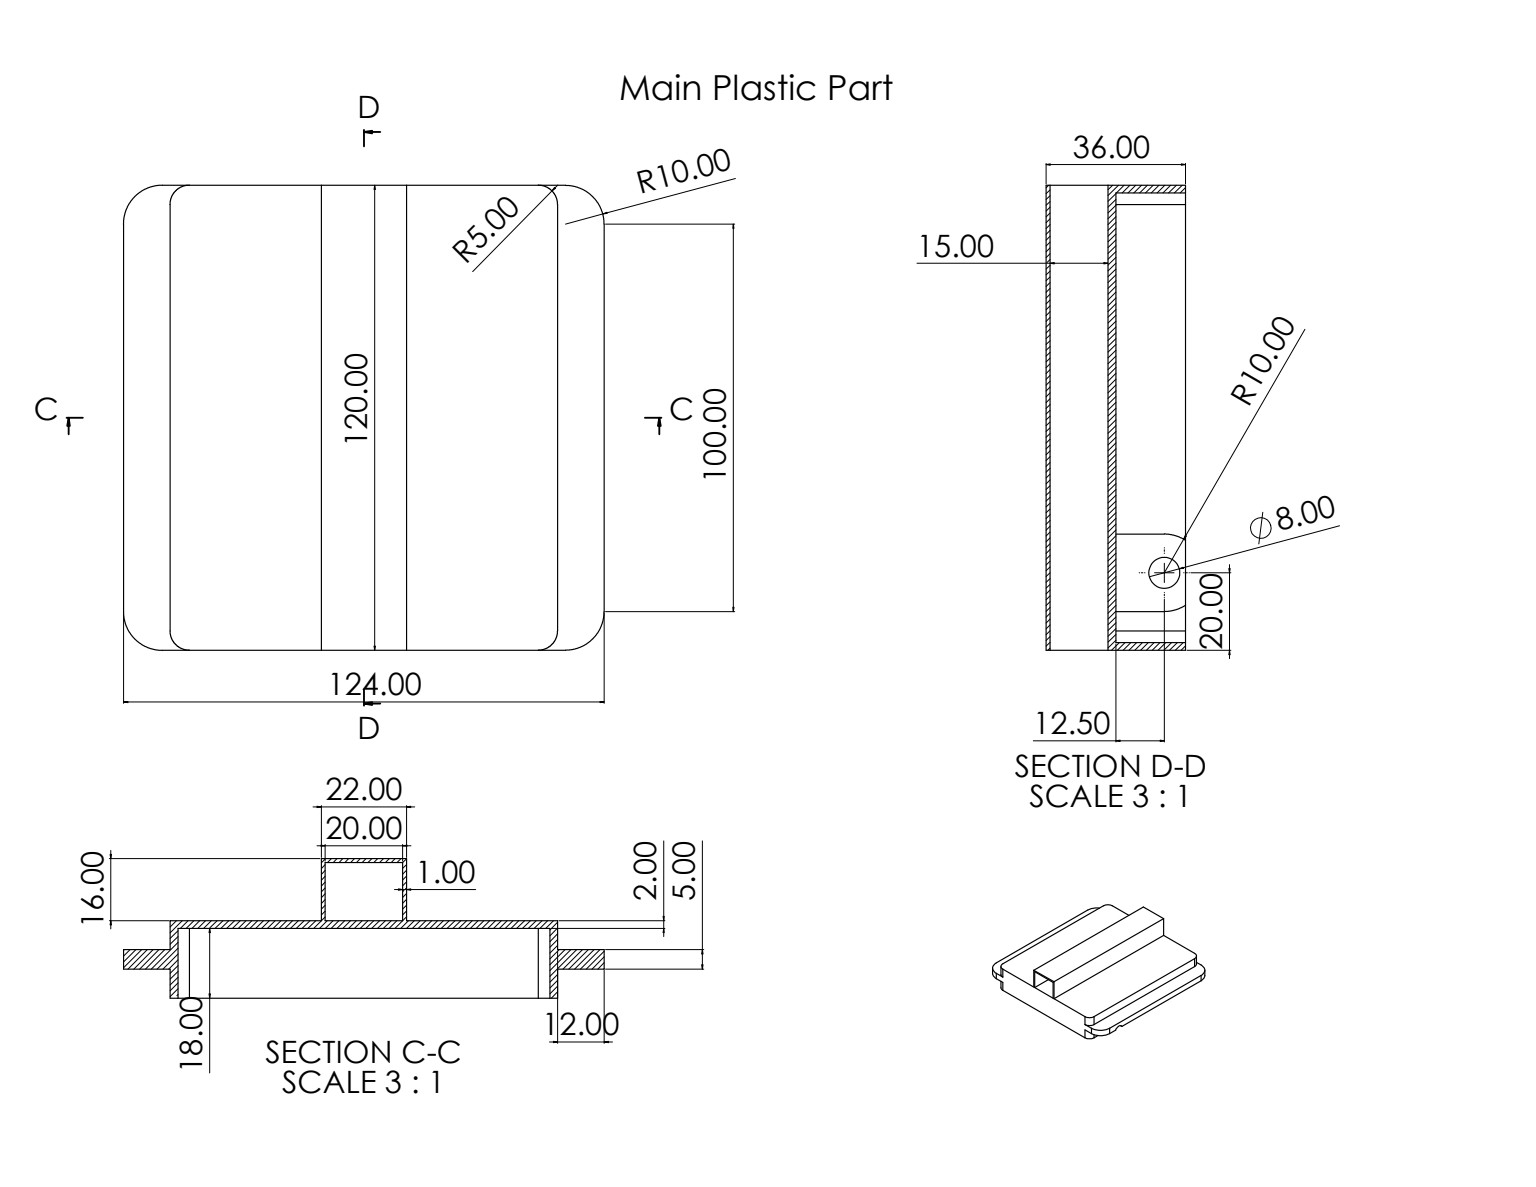
ISO-10303-21;
HEADER;
FILE_DESCRIPTION (('STEP AP214'),
    '1' );
FILE_NAME ('Main Plastic Part.step',
    '2026-10-25T21:42:00',
    ( '' ),
    ( '' ),
    'SwSTEP 2.0',
    'SolidWorks 2025',
    '' );
FILE_SCHEMA (( 'AUTOMOTIVE_DESIGN' ));
ENDSEC;

DATA;
#11=EDGE_CURVE ( 'NONE', #40605, #21661, #7711, .T. ) ;
#16=ORIENTED_EDGE ( 'NONE', *, *, #15282, .F. ) ;
#30=DIRECTION ( 'NONE',  ( 0.000000000000000000, 0.000000000000000000, -1.000000000000000000 ) ) ;
#37=ORIENTED_EDGE ( 'NONE', *, *, #25177, .T. ) ;
#107=ORIENTED_EDGE ( 'NONE', *, *, #6079, .F. ) ;
#112=DIRECTION ( 'NONE',  ( 1.000000000000000000, -0.000000000000000000, -1.067522139062650178E-16 ) ) ;
#115=ORIENTED_EDGE ( 'NONE', *, *, #15723, .T. ) ;
#159=DIRECTION ( 'NONE',  ( 0.000000000000000000, 0.000000000000000000, -1.000000000000000000 ) ) ;
#164=DIRECTION ( 'NONE',  ( -1.000000000000000000, -0.000000000000000000, -0.000000000000000000 ) ) ;
#179=CARTESIAN_POINT ( 'NONE',  ( 10.00000000000000178, 25.00000000000000000, -59.99999999999999289 ) ) ;
#204=ADVANCED_FACE ( 'NONE', ( #16223 ), #3440, .F. ) ;
#231=CARTESIAN_POINT ( 'NONE',  ( 43.18024297220213015, -8.265739277488476588, 38.63781537048668469 ) ) ;
#235=CARTESIAN_POINT ( 'NONE',  ( -50.00000000000001421, -10.00000000000000000, 55.00000000000002132 ) ) ;
#246=DIRECTION ( 'NONE',  ( -0.000000000000000000, -1.000000000000000000, 0.000000000000000000 ) ) ;
#261=ORIENTED_EDGE ( 'NONE', *, *, #37253, .F. ) ;
#327=VECTOR ( 'NONE', #3330, 1000.000000000000000 ) ;
#328=ORIENTED_EDGE ( 'NONE', *, *, #28458, .T. ) ;
#341=PRODUCT_DEFINITION_CONTEXT ( 'detailed design', #12504, 'design' ) ;
#348=CARTESIAN_POINT ( 'NONE',  ( 33.00000000000001421, -10.00000000000000000, 48.35164654424506381 ) ) ;
#443=CARTESIAN_POINT ( 'NONE',  ( 43.17447727835383375, -8.261632567776716840, 41.37333478126254960 ) ) ;
#464=DIRECTION ( 'NONE',  ( 0.000000000000000000, 0.000000000000000000, -1.000000000000000000 ) ) ;
#496=CYLINDRICAL_SURFACE ( 'NONE', #39467, 4.000000000000003553 ) ;
#556=LINE ( 'NONE', #37343, #4887 ) ;
#564=CARTESIAN_POINT ( 'NONE',  ( -62.00000000000002842, -2.499999999999999556, 43.46410161513779258 ) ) ;
#592=ORIENTED_EDGE ( 'NONE', *, *, #4818, .T. ) ;
#604=CARTESIAN_POINT ( 'NONE',  ( 0.000000000000000000, 8.000000000000000000, 0.000000000000000000 ) ) ;
#625=CARTESIAN_POINT ( 'NONE',  ( -62.00000000000002842, -4.500000000000000000, 40.00000000000002842 ) ) ;
#626=VERTEX_POINT ( 'NONE', #3867 ) ;
#638=VECTOR ( 'NONE', #26031, 1000.000000000000000 ) ;
#646=EDGE_CURVE ( 'NONE', #32443, #25917, #5124, .T. ) ;
#653=CARTESIAN_POINT ( 'NONE',  ( 40.70800149128672274, -7.145751311064596933, 37.00000000000002132 ) ) ;
#657=AXIS2_PLACEMENT_3D ( 'NONE', #29066, #36076, #42060 ) ;
#680=LINE ( 'NONE', #26634, #18481 ) ;
#687=DIRECTION ( 'NONE',  ( 1.000000000000000000, 0.000000000000000000, -0.000000000000000000 ) ) ;
#693=ORIENTED_EDGE ( 'NONE', *, *, #31287, .T. ) ;
#729=CARTESIAN_POINT ( 'NONE',  ( 39.50407584885977741, -7.322325674842114829, 42.83643345649426948 ) ) ;
#740=ORIENTED_EDGE ( 'NONE', *, *, #15093, .T. ) ;
#746=VERTEX_POINT ( 'NONE', #11497 ) ;
#774=DIRECTION ( 'NONE',  ( -0.000000000000000000, -0.000000000000000000, 1.000000000000000000 ) ) ;
#779=DIRECTION ( 'NONE',  ( 0.000000000000000000, -1.000000000000000000, 0.000000000000000000 ) ) ;
#795=EDGE_CURVE ( 'NONE', #21937, #903, #18515, .T. ) ;
#798=DIRECTION ( 'NONE',  ( 0.000000000000000000, 0.000000000000000000, -1.000000000000000000 ) ) ;
#806=DIRECTION ( 'NONE',  ( 0.000000000000000000, 1.000000000000000000, 0.000000000000000000 ) ) ;
#808=ORIENTED_EDGE ( 'NONE', *, *, #26182, .F. ) ;
#831=FACE_OUTER_BOUND ( 'NONE', #36369, .T. ) ;
#836=EDGE_LOOP ( 'NONE', ( #19778, #12521, #31733, #1428 ) ) ;
#864=ORIENTED_EDGE ( 'NONE', *, *, #5050, .T. ) ;
#875=AXIS2_PLACEMENT_3D ( 'NONE', #35943, #32748, #35537 ) ;
#895=VERTEX_POINT ( 'NONE', #14657 ) ;
#903=VERTEX_POINT ( 'NONE', #30600 ) ;
#910=VECTOR ( 'NONE', #30254, 1000.000000000000000 ) ;
#912=CARTESIAN_POINT ( 'NONE',  ( -50.00000000000001421, -4.500000000000000000, 40.00000000000002842 ) ) ;
#932=ADVANCED_FACE ( 'NONE', ( #5066, #11042 ), #8259, .F. ) ;
#949=CARTESIAN_POINT ( 'NONE',  ( 38.25871219653468813, -7.965888518254534034, 37.99698286429647709 ) ) ;
#957=ORIENTED_EDGE ( 'NONE', *, *, #37845, .T. ) ;
#962=ORIENTED_EDGE ( 'NONE', *, *, #32421, .T. ) ;
#1024=ORIENTED_EDGE ( 'NONE', *, *, #38610, .T. ) ;
#1025=VERTEX_POINT ( 'NONE', #18250 ) ;
#1029=DIRECTION ( 'NONE',  ( -1.000000000000000000, 0.000000000000000000, 1.067522139062650178E-16 ) ) ;
#1030=EDGE_CURVE ( 'NONE', #9283, #5870, #25406, .T. ) ;
#1040=AXIS2_PLACEMENT_3D ( 'NONE', #31418, #28431, #21630 ) ;
#1104=FACE_OUTER_BOUND ( 'NONE', #28266, .T. ) ;
#1165=FACE_OUTER_BOUND ( 'NONE', #24935, .T. ) ;
#1172=ORIENTED_EDGE ( 'NONE', *, *, #25644, .F. ) ;
#1179=VERTEX_POINT ( 'NONE', #29916 ) ;
#1210=DIRECTION ( 'NONE',  ( 0.000000000000000000, -1.000000000000000000, 0.000000000000000000 ) ) ;
#1211=VERTEX_POINT ( 'NONE', #23115 ) ;
#1217=CARTESIAN_POINT ( 'NONE',  ( -73.31370849898480913, -2.499999999999999556, 36.53589838486226427 ) ) ;
#1223=ORIENTED_EDGE ( 'NONE', *, *, #11786, .T. ) ;
#1232=DIRECTION ( 'NONE',  ( 1.000000000000000000, -0.000000000000000000, 1.156482317317871232E-16 ) ) ;
#1234=ADVANCED_FACE ( 'NONE', ( #19714 ), #38865, .T. ) ;
#1240=AXIS2_PLACEMENT_3D ( 'NONE', #3587, #9987, #2755 ) ;
#1262=EDGE_CURVE ( 'NONE', #27592, #25543, #32683, .T. ) ;
#1265=LINE ( 'NONE', #17638, #24662 ) ;
#1273=DIRECTION ( 'NONE',  ( -1.000000000000000000, 0.000000000000000000, 0.000000000000000000 ) ) ;
#1285=AXIS2_PLACEMENT_3D ( 'NONE', #6696, #16904, #26478 ) ;
#1318=ORIENTED_EDGE ( 'NONE', *, *, #17030, .F. ) ;
#1333=ORIENTED_EDGE ( 'NONE', *, *, #37843, .T. ) ;
#1355=FACE_OUTER_BOUND ( 'NONE', #24355, .T. ) ;
#1363=ORIENTED_EDGE ( 'NONE', *, *, #20185, .T. ) ;
#1366=DIRECTION ( 'NONE',  ( 0.000000000000000000, -1.000000000000000000, 0.000000000000000000 ) ) ;
#1367=CARTESIAN_POINT ( 'NONE',  ( 38.25522726963416176, -7.968137130668702994, 41.99918083815303760 ) ) ;
#1378=ORIENTED_EDGE ( 'NONE', *, *, #10228, .F. ) ;
#1380=VECTOR ( 'NONE', #12567, 1000.000000000000000 ) ;
#1404=CARTESIAN_POINT ( 'NONE',  ( -50.00000000000001421, -10.00000000000000000, -59.99999999999999289 ) ) ;
#1428=ORIENTED_EDGE ( 'NONE', *, *, #13150, .T. ) ;
#1429=VERTEX_POINT ( 'NONE', #23010 ) ;
#1442=CARTESIAN_POINT ( 'NONE',  ( -11.00000000000000355, 26.00000000000000355, -87.20294101747086302 ) ) ;
#1449=VECTOR ( 'NONE', #35176, 1000.000000000000000 ) ;
#1458=CARTESIAN_POINT ( 'NONE',  ( 10.00000000000000178, 10.00000000000000000, -87.20294101747086302 ) ) ;
#1462=CARTESIAN_POINT ( 'NONE',  ( -50.00000000000001421, -10.00000000000000000, 60.00000000000002132 ) ) ;
#1487=CARTESIAN_POINT ( 'NONE',  ( 11.00000000000000355, 26.00000000000000355, 60.00000000000002132 ) ) ;
#1489=EDGE_CURVE ( 'NONE', #27620, #7819, #28127, .T. ) ;
#1495=VECTOR ( 'NONE', #26536, 1000.000000000000000 ) ;
#1517=VECTOR ( 'NONE', #35936, 1000.000000000000000 ) ;
#1578=CARTESIAN_POINT ( 'NONE',  ( -45.00000000000002132, -10.00000000000000000, 55.00000000000002132 ) ) ;
#1612=AXIS2_PLACEMENT_3D ( 'NONE', #37044, #41057, #34256 ) ;
#1632=VECTOR ( 'NONE', #15338, 1000.000000000000000 ) ;
#1645=VECTOR ( 'NONE', #12236, 1000.000000000000000 ) ;
#1727=DIRECTION ( 'NONE',  ( -0.000000000000000000, 1.000000000000000000, 0.000000000000000000 ) ) ;
#1804=CARTESIAN_POINT ( 'NONE',  ( -73.31370849898480913, -2.499999999999999556, 43.46410161513779258 ) ) ;
#1841=VERTEX_POINT ( 'NONE', #34471 ) ;
#1862=CARTESIAN_POINT ( 'NONE',  ( 0.000000000000000000, -10.00000000000000000, 0.000000000000000000 ) ) ;
#1895=ORIENTED_EDGE ( 'NONE', *, *, #12828, .F. ) ;
#1906=DIRECTION ( 'NONE',  ( 1.000000000000000000, 0.000000000000000000, -1.067522139062650302E-16 ) ) ;
#1945=EDGE_CURVE ( 'NONE', #33276, #24557, #9582, .T. ) ;
#1986=CARTESIAN_POINT ( 'NONE',  ( 10.00000000000000178, 25.00000000000000000, 60.00000000000002132 ) ) ;
#2006=LINE ( 'NONE', #22407, #638 ) ;
#2034=EDGE_CURVE ( 'NONE', #21661, #9431, #36574, .T. ) ;
#2045=EDGE_LOOP ( 'NONE', ( #33378, #14401, #40294, #13987, #23060, #23283, #39786, #27182 ) ) ;
#2069=CARTESIAN_POINT ( 'NONE',  ( 44.99999999999999289, -10.00000000000000000, 55.00000000000002132 ) ) ;
#2087=CARTESIAN_POINT ( 'NONE',  ( 47.99999999999998579, 10.00000000000000000, 55.00000000000002132 ) ) ;
#2100=AXIS2_PLACEMENT_3D ( 'NONE', #11181, #7782, #14788 ) ;
#2110=ORIENTED_EDGE ( 'NONE', *, *, #28530, .T. ) ;
#2134=CARTESIAN_POINT ( 'NONE',  ( 52.00000000000002842, 2.499999999999999556, 50.00000000000001421 ) ) ;
#2137=DIRECTION ( 'NONE',  ( -1.000000000000000000, 0.000000000000000000, 0.000000000000000000 ) ) ;
#2148=CARTESIAN_POINT ( 'NONE',  ( -48.00000000000001421, 8.000000000000000000, 55.00000000000002132 ) ) ;
#2161=ORIENTED_EDGE ( 'NONE', *, *, #14749, .T. ) ;
#2180=DIRECTION ( 'NONE',  ( 0.000000000000000000, 0.000000000000000000, -1.000000000000000000 ) ) ;
#2206=AXIS2_PLACEMENT_3D ( 'NONE', #34511, #5369, #18348 ) ;
#2215=CARTESIAN_POINT ( 'NONE',  ( 40.50000000000000711, -15.00000000000000000, 37.00000000000001421 ) ) ;
#2246=ORIENTED_EDGE ( 'NONE', *, *, #5463, .T. ) ;
#2251=DIRECTION ( 'NONE',  ( 1.000000000000000000, -0.000000000000000000, -0.000000000000000000 ) ) ;
#2306=LINE ( 'NONE', #8897, #20278 ) ;
#2317=DIRECTION ( 'NONE',  ( 0.000000000000000000, -0.000000000000000000, 1.000000000000000000 ) ) ;
#2367=FACE_OUTER_BOUND ( 'NONE', #20004, .T. ) ;
#2378=CARTESIAN_POINT ( 'NONE',  ( -45.00000000000002132, 10.00000000000000000, -59.99999999999999289 ) ) ;
#2410=CYLINDRICAL_SURFACE ( 'NONE', #20954, 10.00000000000000178 ) ;
#2431=CARTESIAN_POINT ( 'NONE',  ( 44.99999999999998579, -2.499999999999999556, -60.00000000000000000 ) ) ;
#2449=CARTESIAN_POINT ( 'NONE',  ( -52.00000000000002842, 10.00000000000000000, 50.00000000000001421 ) ) ;
#2466=ADVANCED_FACE ( 'NONE', ( #16576 ), #26563, .T. ) ;
#2475=PLANE ( 'NONE',  #25989 ) ;
#2479=ORIENTED_EDGE ( 'NONE', *, *, #10263, .F. ) ;
#2484=ADVANCED_FACE ( 'NONE', ( #3797 ), #10612, .T. ) ;
#2587=EDGE_CURVE ( 'NONE', #21661, #40605, #5052, .T. ) ;
#2637=AXIS2_PLACEMENT_3D ( 'NONE', #3251, #24973, #19416 ) ;
#2655=DIRECTION ( 'NONE',  ( -0.000000000000000000, -1.000000000000000000, -0.000000000000000000 ) ) ;
#2662=ORIENTED_EDGE ( 'NONE', *, *, #4575, .F. ) ;
#2673=VECTOR ( 'NONE', #26163, 1000.000000000000000 ) ;
#2681=EDGE_LOOP ( 'NONE', ( #33551, #6500, #40081, #37 ) ) ;
#2683=DIRECTION ( 'NONE',  ( -1.000000000000000000, 0.000000000000000000, 0.000000000000000000 ) ) ;
#2688=ORIENTED_EDGE ( 'NONE', *, *, #23153, .T. ) ;
#2700=PLANE ( 'NONE',  #28201 ) ;
#2715=EDGE_LOOP ( 'NONE', ( #328, #26233, #27210, #38333, #36525 ) ) ;
#2716=VECTOR ( 'NONE', #28782, 1000.000000000000000 ) ;
#2725=EDGE_CURVE ( 'NONE', #27773, #37476, #17421, .T. ) ;
#2755=DIRECTION ( 'NONE',  ( 0.000000000000000000, -0.000000000000000000, -1.000000000000000000 ) ) ;
#2769=VERTEX_POINT ( 'NONE', #21018 ) ;
#2789=AXIS2_PLACEMENT_3D ( 'NONE', #41130, #18160, #37931 ) ;
#2794=ORIENTED_EDGE ( 'NONE', *, *, #12455, .T. ) ;
#2825=ORIENTED_EDGE ( 'NONE', *, *, #37937, .F. ) ;
#2828=DIRECTION ( 'NONE',  ( 0.000000000000000000, 0.000000000000000000, -1.000000000000000000 ) ) ;
#2836=ORIENTED_EDGE ( 'NONE', *, *, #40187, .T. ) ;
#2839=ORIENTED_EDGE ( 'NONE', *, *, #2725, .F. ) ;
#2857=DIRECTION ( 'NONE',  ( 1.000000000000000000, -0.000000000000000000, -1.067522139062650178E-16 ) ) ;
#2878=PLANE ( 'NONE',  #12962 ) ;
#2894=FACE_OUTER_BOUND ( 'NONE', #8992, .T. ) ;
#2895=LINE ( 'NONE', #38623, #28106 ) ;
#2907=AXIS2_PLACEMENT_3D ( 'NONE', #17046, #10238, #16835 ) ;
#2971=VECTOR ( 'NONE', #4498, 1000.000000000000000 ) ;
#2990=CARTESIAN_POINT ( 'NONE',  ( -33.00000000000001421, 8.000000000000000000, 50.00000000000002842 ) ) ;
#3019=CARTESIAN_POINT ( 'NONE',  ( 40.50000000000000711, -15.00000000000000000, 40.00000000000002842 ) ) ;
#3101=ORIENTED_EDGE ( 'NONE', *, *, #4888, .T. ) ;
#3104=VERTEX_POINT ( 'NONE', #39473 ) ;
#3107=ORIENTED_EDGE ( 'NONE', *, *, #19744, .T. ) ;
#3118=EDGE_CURVE ( 'NONE', #1025, #28880, #3333, .T. ) ;
#3124=ADVANCED_BREP_SHAPE_REPRESENTATION ( '', ( #10332, #40442 ), #28197 ) ;
#3135=CYLINDRICAL_SURFACE ( 'NONE', #26509, 4.999999999999997335 ) ;
#3142=DIRECTION ( 'NONE',  ( 1.000000000000000000, 0.000000000000000000, -0.000000000000000000 ) ) ;
#3239=DIRECTION ( 'NONE',  ( 0.000000000000000000, -0.000000000000000000, -1.000000000000000000 ) ) ;
#3251=CARTESIAN_POINT ( 'NONE',  ( -50.00000000000001421, 10.00000000000000000, -57.99999999999998579 ) ) ;
#3291=VERTEX_POINT ( 'NONE', #20968 ) ;
#3308=ORIENTED_EDGE ( 'NONE', *, *, #21156, .T. ) ;
#3330=DIRECTION ( 'NONE',  ( -1.156482317317871232E-16, -0.000000000000000000, -1.000000000000000000 ) ) ;
#3333=LINE ( 'NONE', #348, #26173 ) ;
#3357=DIRECTION ( 'NONE',  ( -0.000000000000000000, 1.000000000000000000, -0.000000000000000000 ) ) ;
#3363=FACE_OUTER_BOUND ( 'NONE', #31140, .T. ) ;
#3365=ORIENTED_EDGE ( 'NONE', *, *, #27211, .F. ) ;
#3393=LINE ( 'NONE', #13177, #2673 ) ;
#3402=ORIENTED_EDGE ( 'NONE', *, *, #25736, .T. ) ;
#3423=CARTESIAN_POINT ( 'NONE',  ( 43.47980401598100286, -8.484779524062236788, 39.59649023839028814 ) ) ;
#3440=PLANE ( 'NONE',  #15889 ) ;
#3444=CARTESIAN_POINT ( 'NONE',  ( 44.99999999999999289, 8.000000000000000000, 55.00000000000002132 ) ) ;
#3451=ORIENTED_EDGE ( 'NONE', *, *, #9825, .F. ) ;
#3453=AXIS2_PLACEMENT_3D ( 'NONE', #11912, #21494, #28289 ) ;
#3481=CARTESIAN_POINT ( 'NONE',  ( 62.00000000000002842, -2.499999999999999556, 43.46410161513777837 ) ) ;
#3488=CARTESIAN_POINT ( 'NONE',  ( -45.00000000000002132, 2.499999999999999556, -55.00000000000000000 ) ) ;
#3502=ORIENTED_EDGE ( 'NONE', *, *, #30309, .T. ) ;
#3519=VECTOR ( 'NONE', #774, 1000.000000000000000 ) ;
#3537=FACE_OUTER_BOUND ( 'NONE', #7186, .T. ) ;
#3541=DIRECTION ( 'NONE',  ( 0.000000000000000000, 0.000000000000000000, -1.000000000000000000 ) ) ;
#3572=CARTESIAN_POINT ( 'NONE',  ( -9.999999999999998224, 25.00000000000000000, -59.99999999999999289 ) ) ;
#3587=CARTESIAN_POINT ( 'NONE',  ( 40.50000000000000711, -15.00000000000000000, 40.00000000000002842 ) ) ;
#3630=EDGE_CURVE ( 'NONE', #16152, #5136, #7024, .T. ) ;
#3636=CARTESIAN_POINT ( 'NONE',  ( 49.99999999999998579, 10.00000000000000000, 60.00000000000002132 ) ) ;
#3669=CARTESIAN_POINT ( 'NONE',  ( -52.00000000000002842, -2.500000000000000444, 50.00000000000001421 ) ) ;
#3698=FACE_OUTER_BOUND ( 'NONE', #32650, .T. ) ;
#3718=DIRECTION ( 'NONE',  ( 0.000000000000000000, 0.000000000000000000, 1.000000000000000000 ) ) ;
#3741=DIRECTION ( 'NONE',  ( -0.000000000000000000, -1.000000000000000000, -0.000000000000000000 ) ) ;
#3797=FACE_OUTER_BOUND ( 'NONE', #34218, .T. ) ;
#3799=EDGE_CURVE ( 'NONE', #36692, #33611, #25470, .T. ) ;
#3807=EDGE_CURVE ( 'NONE', #2769, #16441, #13220, .T. ) ;
#3813=DIRECTION ( 'NONE',  ( -1.000000000000000000, 0.000000000000000000, 0.000000000000000000 ) ) ;
#3820=ORIENTED_EDGE ( 'NONE', *, *, #28458, .F. ) ;
#3821=DIRECTION ( 'NONE',  ( -0.000000000000000000, 1.000000000000000000, -0.000000000000000000 ) ) ;
#3829=VERTEX_POINT ( 'NONE', #17468 ) ;
#3847=CARTESIAN_POINT ( 'NONE',  ( 40.50000000000000711, -7.145751311064572064, 43.00000000000004263 ) ) ;
#3867=CARTESIAN_POINT ( 'NONE',  ( -49.99999999999998579, -2.499999999999999556, 43.46410161513779258 ) ) ;
#3884=CARTESIAN_POINT ( 'NONE',  ( -33.00000000000001421, -4.499999999999999112, 44.00000000000003553 ) ) ;
#3926=VERTEX_POINT ( 'NONE', #16167 ) ;
#3936=ORIENTED_EDGE ( 'NONE', *, *, #37619, .F. ) ;
#3956=LINE ( 'NONE', #36284, #3519 ) ;
#3973=CARTESIAN_POINT ( 'NONE',  ( 44.99999999999998579, 2.499999999999999556, 60.00000000000002132 ) ) ;
#3988=ORIENTED_EDGE ( 'NONE', *, *, #15039, .F. ) ;
#4007=CARTESIAN_POINT ( 'NONE',  ( -50.00000000000001421, 10.00000000000000000, 60.00000000000002132 ) ) ;
#4030=VERTEX_POINT ( 'NONE', #5737 ) ;
#4057=CIRCLE ( 'NONE', #16977, 4.000000000000003553 ) ;
#4075=CIRCLE ( 'NONE', #38684, 4.000000000000003553 ) ;
#4121=AXIS2_PLACEMENT_3D ( 'NONE', #36302, #39490, #10579 ) ;
#4126=ADVANCED_FACE ( 'NONE', ( #19969 ), #6577, .F. ) ;
#4135=VERTEX_POINT ( 'NONE', #32936 ) ;
#4205=CARTESIAN_POINT ( 'NONE',  ( -62.00000000000001421, 2.499999999999999556, -60.00000000000000000 ) ) ;
#4209=CARTESIAN_POINT ( 'NONE',  ( -73.31370849898480913, -2.499999999999999556, 43.46410161513779258 ) ) ;
#4217=CIRCLE ( 'NONE', #27986, 10.00000000000000178 ) ;
#4222=DIRECTION ( 'NONE',  ( 0.000000000000000000, -1.000000000000000000, 0.000000000000000000 ) ) ;
#4284=CARTESIAN_POINT ( 'NONE',  ( -33.00000000000001421, -4.500000000000000000, 30.00000000000002842 ) ) ;
#4329=VECTOR ( 'NONE', #2137, 1000.000000000000000 ) ;
#4337=EDGE_CURVE ( 'NONE', #26542, #37769, #27538, .T. ) ;
#4345=CARTESIAN_POINT ( 'NONE',  ( 37.60297877579395021, -8.423259317252886902, 40.80592701207748974 ) ) ;
#4359=ORIENTED_EDGE ( 'NONE', *, *, #40890, .F. ) ;
#4383=CARTESIAN_POINT ( 'NONE',  ( 33.00000000000001421, -4.500000000000000888, 50.00000000000002842 ) ) ;
#4450=CARTESIAN_POINT ( 'NONE',  ( 49.99999999999998579, -2.499999999999999556, -54.99999999999997158 ) ) ;
#4463=ORIENTED_EDGE ( 'NONE', *, *, #1945, .T. ) ;
#4465=CARTESIAN_POINT ( 'NONE',  ( 44.99999999999998579, 2.499999999999999556, -60.00000000000000000 ) ) ;
#4498=DIRECTION ( 'NONE',  ( -0.000000000000000000, -1.000000000000000000, 0.000000000000000000 ) ) ;
#4537=CARTESIAN_POINT ( 'NONE',  ( 47.99999999999998579, 8.000000000000000000, -54.99999999999997158 ) ) ;
#4548=CARTESIAN_POINT ( 'NONE',  ( 49.99999999999998579, 10.00000000000000000, 55.00000000000002132 ) ) ;
#4575=EDGE_CURVE ( 'NONE', #41347, #30811, #12582, .T. ) ;
#4591=CARTESIAN_POINT ( 'NONE',  ( 11.00000000000000355, 26.00000000000000355, -87.20294101747086302 ) ) ;
#4617=ORIENTED_EDGE ( 'NONE', *, *, #36365, .F. ) ;
#4626=CARTESIAN_POINT ( 'NONE',  ( -45.00000000000002132, -2.499999999999999556, 55.00000000000002132 ) ) ;
#4634=EDGE_CURVE ( 'NONE', #26169, #21937, #40928, .T. ) ;
#4651=DIRECTION ( 'NONE',  ( 0.000000000000000000, 0.000000000000000000, -1.000000000000000000 ) ) ;
#4725=EDGE_CURVE ( 'NONE', #2769, #15408, #8600, .T. ) ;
#4775=VECTOR ( 'NONE', #18902, 1000.000000000000000 ) ;
#4782=DIRECTION ( 'NONE',  ( -1.000000000000000000, 0.000000000000000000, 0.000000000000000000 ) ) ;
#4814=ADVANCED_FACE ( 'NONE', ( #15416 ), #28368, .T. ) ;
#4818=EDGE_CURVE ( 'NONE', #21965, #16039, #7982, .T. ) ;
#4822=VERTEX_POINT ( 'NONE', #27553 ) ;
#4854=CARTESIAN_POINT ( 'NONE',  ( -45.00000000000002132, 10.00000000000000000, 60.00000000000002132 ) ) ;
#4869=DIRECTION ( 'NONE',  ( 0.000000000000000000, 0.000000000000000000, -1.000000000000000000 ) ) ;
#4870=VECTOR ( 'NONE', #4222, 1000.000000000000000 ) ;
#4876=ORIENTED_EDGE ( 'NONE', *, *, #41025, .F. ) ;
#4887=VECTOR ( 'NONE', #31159, 1000.000000000000000 ) ;
#4888=EDGE_CURVE ( 'NONE', #13780, #1025, #19868, .T. ) ;
#4895=DIRECTION ( 'NONE',  ( 0.000000000000000000, -1.000000000000000000, 0.000000000000000000 ) ) ;
#4933=CIRCLE ( 'NONE', #29356, 3.000000000000016431 ) ;
#4936=( GEOMETRIC_REPRESENTATION_CONTEXT ( 3 ) GLOBAL_UNCERTAINTY_ASSIGNED_CONTEXT ( ( #22893 ) ) GLOBAL_UNIT_ASSIGNED_CONTEXT ( ( #10878, #34252, #34457 ) ) REPRESENTATION_CONTEXT ( 'NONE', 'WORKASPACE' ) );
#5006=FACE_OUTER_BOUND ( 'NONE', #29572, .T. ) ;
#5009=CARTESIAN_POINT ( 'NONE',  ( -45.00000000000002132, 8.000000000000000000, 55.00000000000002132 ) ) ;
#5028=ORIENTED_EDGE ( 'NONE', *, *, #16775, .T. ) ;
#5050=EDGE_CURVE ( 'NONE', #21937, #9969, #31032, .T. ) ;
#5052=CIRCLE ( 'NONE', #21363, 4.000000000000010658 ) ;
#5060=DIRECTION ( 'NONE',  ( -0.000000000000000000, -0.000000000000000000, 1.000000000000000000 ) ) ;
#5066=FACE_BOUND ( 'NONE', #5614, .T. ) ;
#5069=DIRECTION ( 'NONE',  ( -1.000000000000000000, 0.000000000000000000, 0.000000000000000000 ) ) ;
#5072=DIRECTION ( 'NONE',  ( -0.000000000000000000, 1.000000000000000000, -0.000000000000000000 ) ) ;
#5084=ORIENTED_EDGE ( 'NONE', *, *, #17030, .T. ) ;
#5104=DIRECTION ( 'NONE',  ( 0.000000000000000000, -1.000000000000000000, 0.000000000000000000 ) ) ;
#5124=LINE ( 'NONE', #30657, #4329 ) ;
#5136=VERTEX_POINT ( 'NONE', #12729 ) ;
#5151=CARTESIAN_POINT ( 'NONE',  ( 49.99999999999998579, -10.00000000000000000, 55.00000000000002132 ) ) ;
#5173=APPLICATION_CONTEXT ( 'automotive_design' ) ;
#5201=CARTESIAN_POINT ( 'NONE',  ( 52.00000000000002132, 2.499999999999999556, -60.00000000000000000 ) ) ;
#5222=DIRECTION ( 'NONE',  ( 0.000000000000000000, 0.000000000000000000, -1.000000000000000000 ) ) ;
#5227=ORIENTED_EDGE ( 'NONE', *, *, #5949, .T. ) ;
#5259=ORIENTED_EDGE ( 'NONE', *, *, #38952, .F. ) ;
#5277=ORIENTED_EDGE ( 'NONE', *, *, #8224, .T. ) ;
#5281=CARTESIAN_POINT ( 'NONE',  ( 52.00000000000002132, 10.00000000000000000, 60.00000000000002132 ) ) ;
#5294=VERTEX_POINT ( 'NONE', #26545 ) ;
#5295=CARTESIAN_POINT ( 'NONE',  ( 62.00000000000002842, -2.499999999999999556, 36.53589838486225005 ) ) ;
#5369=DIRECTION ( 'NONE',  ( 0.000000000000000000, -1.000000000000000000, 0.000000000000000000 ) ) ;
#5399=CIRCLE ( 'NONE', #31206, 4.999999999999984013 ) ;
#5421=DIRECTION ( 'NONE',  ( 0.000000000000000000, 0.000000000000000000, 1.000000000000000000 ) ) ;
#5463=EDGE_CURVE ( 'NONE', #36810, #626, #12646, .T. ) ;
#5472=FACE_BOUND ( 'NONE', #38192, .T. ) ;
#5480=CYLINDRICAL_SURFACE ( 'NONE', #657, 10.00000000000000178 ) ;
#5490=LINE ( 'NONE', #21649, #16316 ) ;
#5495=PLANE ( 'NONE',  #29429 ) ;
#5504=VERTEX_POINT ( 'NONE', #27512 ) ;
#5505=AXIS2_PLACEMENT_3D ( 'NONE', #41572, #15628, #31987 ) ;
#5510=EDGE_LOOP ( 'NONE', ( #34428, #8429, #12576, #23384, #26391, #957 ) ) ;
#5514=ORIENTED_EDGE ( 'NONE', *, *, #23156, .F. ) ;
#5523=DIRECTION ( 'NONE',  ( 0.000000000000000000, 0.000000000000000000, -1.000000000000000000 ) ) ;
#5531=CARTESIAN_POINT ( 'NONE',  ( -48.00000000000001421, -10.00000000000000000, 0.000000000000000000 ) ) ;
#5541=CARTESIAN_POINT ( 'NONE',  ( 33.00000000000001421, 7.999999999999996447, 50.00000000000002842 ) ) ;
#5554=ORIENTED_EDGE ( 'NONE', *, *, #4818, .F. ) ;
#5569=VERTEX_POINT ( 'NONE', #4537 ) ;
#5577=AXIS2_PLACEMENT_3D ( 'NONE', #41442, #8680, #40805 ) ;
#5614=EDGE_LOOP ( 'NONE', ( #35753, #962, #592, #7959 ) ) ;
#5622=CARTESIAN_POINT ( 'NONE',  ( 33.00000000000001421, 8.000000000000000000, 30.00000000000002132 ) ) ;
#5635=DIRECTION ( 'NONE',  ( 0.000000000000000000, 0.000000000000000000, -1.000000000000000000 ) ) ;
#5675=DIRECTION ( 'NONE',  ( -1.000000000000000000, -0.000000000000000000, -0.000000000000000000 ) ) ;
#5722=DIRECTION ( 'NONE',  ( 1.000000000000000000, 0.000000000000000000, 0.000000000000000000 ) ) ;
#5737=CARTESIAN_POINT ( 'NONE',  ( 40.50000000000000711, -15.00000000000000000, 43.00000000000004263 ) ) ;
#5744=DIRECTION ( 'NONE',  ( 0.000000000000000000, 0.000000000000000000, 1.000000000000000000 ) ) ;
#5831=DIRECTION ( 'NONE',  ( 0.000000000000000000, 0.000000000000000000, 1.000000000000000000 ) ) ;
#5843=DIRECTION ( 'NONE',  ( 0.000000000000000000, -0.000000000000000000, 1.000000000000000000 ) ) ;
#5869=ORIENTED_EDGE ( 'NONE', *, *, #15630, .F. ) ;
#5870=VERTEX_POINT ( 'NONE', #40679 ) ;
#5872=VERTEX_POINT ( 'NONE', #11535 ) ;
#5879=EDGE_CURVE ( 'NONE', #7445, #3104, #24528, .T. ) ;
#5881=LINE ( 'NONE', #18852, #10213 ) ;
#5894=CYLINDRICAL_SURFACE ( 'NONE', #1040, 3.000000000000002665 ) ;
#5895=DIRECTION ( 'NONE',  ( -2.312964634635743450E-16, -1.000000000000000000, 0.000000000000000000 ) ) ;
#5913=EDGE_CURVE ( 'NONE', #16441, #5294, #35556, .T. ) ;
#5949=EDGE_CURVE ( 'NONE', #17804, #4030, #4933, .T. ) ;
#5968=ORIENTED_EDGE ( 'NONE', *, *, #23242, .F. ) ;
#6005=CARTESIAN_POINT ( 'NONE',  ( 44.99999999999998579, 2.499999999999999556, -60.00000000000000000 ) ) ;
#6046=CARTESIAN_POINT ( 'NONE',  ( -73.31370849898480913, -4.500000000000000000, 40.00000000000002842 ) ) ;
#6074=VERTEX_POINT ( 'NONE', #26403 ) ;
#6079=EDGE_CURVE ( 'NONE', #28880, #41347, #22166, .T. ) ;
#6097=DIRECTION ( 'NONE',  ( 0.000000000000000000, 0.000000000000000000, -1.000000000000000000 ) ) ;
#6108=DIRECTION ( 'NONE',  ( 0.000000000000000000, 0.000000000000000000, -1.000000000000000000 ) ) ;
#6133=ORIENTED_EDGE ( 'NONE', *, *, #29983, .T. ) ;
#6143=VERTEX_POINT ( 'NONE', #235 ) ;
#6159=EDGE_CURVE ( 'NONE', #27680, #1179, #19588, .T. ) ;
#6173=CIRCLE ( 'NONE', #2100, 4.000000000000010658 ) ;
#6225=DIRECTION ( 'NONE',  ( -0.000000000000000000, 1.000000000000000000, -0.000000000000000000 ) ) ;
#6247=AXIS2_PLACEMENT_3D ( 'NONE', #4205, #1232, #14201 ) ;
#6260=VECTOR ( 'NONE', #33757, 1000.000000000000000 ) ;
#6308=VECTOR ( 'NONE', #13831, 1000.000000000000000 ) ;
#6408=ORIENTED_EDGE ( 'NONE', *, *, #36192, .F. ) ;
#6425=ORIENTED_EDGE ( 'NONE', *, *, #3630, .F. ) ;
#6427=CARTESIAN_POINT ( 'NONE',  ( 47.99999999999998579, -10.00000000000000000, -54.99999999999997158 ) ) ;
#6442=ADVANCED_FACE ( 'NONE', ( #27654 ), #24687, .F. ) ;
#6467=CARTESIAN_POINT ( 'NONE',  ( 44.99999999999998579, 10.00000000000000000, 58.00000000000001421 ) ) ;
#6488=ORIENTED_EDGE ( 'NONE', *, *, #15512, .F. ) ;
#6500=ORIENTED_EDGE ( 'NONE', *, *, #36192, .T. ) ;
#6526=VECTOR ( 'NONE', #11836, 1000.000000000000000 ) ;
#6527=CARTESIAN_POINT ( 'NONE',  ( 62.00000000000001421, -2.499999999999999556, -60.00000000000000000 ) ) ;
#6550=DIRECTION ( 'NONE',  ( -1.000000000000000000, 0.000000000000000000, 0.000000000000000000 ) ) ;
#6577=PLANE ( 'NONE',  #8483 ) ;
#6606=ADVANCED_FACE ( 'NONE', ( #9568, #22317 ), #13169, .T. ) ;
#6615=VERTEX_POINT ( 'NONE', #29317 ) ;
#6653=LINE ( 'NONE', #15827, #30584 ) ;
#6654=ORIENTED_EDGE ( 'NONE', *, *, #32421, .F. ) ;
#6683=ADVANCED_FACE ( 'NONE', ( #17213 ), #30176, .T. ) ;
#6691=DIRECTION ( 'NONE',  ( 0.000000000000000000, 0.000000000000000000, -1.000000000000000000 ) ) ;
#6696=CARTESIAN_POINT ( 'NONE',  ( -50.00000000000001421, 10.00000000000000000, 60.00000000000002132 ) ) ;
#6706=CARTESIAN_POINT ( 'NONE',  ( 40.50000000000000711, -15.00000000000000000, 40.00000000000002842 ) ) ;
#6733=DIRECTION ( 'NONE',  ( 0.000000000000000000, 0.000000000000000000, 1.000000000000000000 ) ) ;
#6737=AXIS2_PLACEMENT_3D ( 'NONE', #625, #13602, #26586 ) ;
#6767=AXIS2_PLACEMENT_3D ( 'NONE', #3444, #6225, #464 ) ;
#6796=AXIS2_PLACEMENT_3D ( 'NONE', #3488, #35408, #22645 ) ;
#6804=VERTEX_POINT ( 'NONE', #18349 ) ;
#6822=CARTESIAN_POINT ( 'NONE',  ( 42.47436581990372417, -7.799571033938490494, 42.26655061162645666 ) ) ;
#6834=PLANE ( 'NONE',  #41023 ) ;
#6925=EDGE_CURVE ( 'NONE', #3829, #13352, #37712, .T. ) ;
#6941=VECTOR ( 'NONE', #34630, 1000.000000000000000 ) ;
#6946=AXIS2_PLACEMENT_3D ( 'NONE', #37929, #28142, #41128 ) ;
#6959=CARTESIAN_POINT ( 'NONE',  ( -45.00000000000002132, 8.000000000000000000, -57.99999999999998579 ) ) ;
#6965=EDGE_CURVE ( 'NONE', #40353, #2769, #33518, .T. ) ;
#6968=EDGE_LOOP ( 'NONE', ( #24384, #11262 ) ) ;
#7003=PLANE ( 'NONE',  #10442 ) ;
#7017=ORIENTED_EDGE ( 'NONE', *, *, #25999, .T. ) ;
#7023=DIRECTION ( 'NONE',  ( 0.000000000000000000, 0.000000000000000000, -1.000000000000000000 ) ) ;
#7024=B_SPLINE_CURVE_WITH_KNOTS ( 'NONE', 3,
 ( #3847, #13414, #20015, #39794, #29579, #16619, #16416, #40000, #6822, #32763, #10867, #10659, #443, #23639, #7037, #32980, #36388, #29362, #3423, #39349, #23854, #231, #36819, #32556, #16826, #13213, #13844, #17038, #29789, #26399, #26199, #10029, #653, #22990 ),
 .UNSPECIFIED., .F., .F.,
 ( 4, 2, 2, 2, 2, 2, 2, 2, 2, 2, 2, 2, 2, 2, 2, 2, 4 ),
 ( 0.009798846907125863953, 0.01041007677969117695, 0.01102130665225648995, 0.01163253652482180295, 0.01224376639738711595, 0.01285499626995243068, 0.01346622614251774541, 0.01407745601508305841, 0.01468868588764837314, 0.01529991576021368788, 0.01591114563277900087, 0.01652237550534431387, 0.01713360537790963034, 0.01774483525047494334, 0.01835606512304025634, 0.01896729499560556934, 0.01957852486817088233 ),
 .UNSPECIFIED. ) ;
#7030=ORIENTED_EDGE ( 'NONE', *, *, #16395, .T. ) ;
#7033=VECTOR ( 'NONE', #22119, 1000.000000000000000 ) ;
#7037=CARTESIAN_POINT ( 'NONE',  ( 43.39384097729021761, -8.420909710220554345, 40.81658779571956330 ) ) ;
#7084=DIRECTION ( 'NONE',  ( 0.000000000000000000, -1.000000000000000000, 0.000000000000000000 ) ) ;
#7086=( LENGTH_UNIT ( ) NAMED_UNIT ( * ) SI_UNIT ( .MILLI., .METRE. ) );
#7114=DIRECTION ( 'NONE',  ( 1.000000000000000000, 0.000000000000000000, 0.000000000000000000 ) ) ;
#7131=DIRECTION ( 'NONE',  ( -0.000000000000000000, -1.000000000000000000, -0.000000000000000000 ) ) ;
#7154=VECTOR ( 'NONE', #34546, 1000.000000000000000 ) ;
#7186=EDGE_LOOP ( 'NONE', ( #2825, #19657, #18734, #10003 ) ) ;
#7195=ORIENTED_EDGE ( 'NONE', *, *, #5463, .F. ) ;
#7339=DIRECTION ( 'NONE',  ( 1.000000000000000000, 0.000000000000000000, 0.000000000000000000 ) ) ;
#7344=ORIENTED_EDGE ( 'NONE', *, *, #30994, .T. ) ;
#7357=CARTESIAN_POINT ( 'NONE',  ( 52.00000000000002132, 10.00000000000000000, -59.99999999999999289 ) ) ;
#7383=LINE ( 'NONE', #13771, #15085 ) ;
#7386=CARTESIAN_POINT ( 'NONE',  ( 47.99999999999999289, -10.00000000000000000, 55.00000000000002132 ) ) ;
#7411=AXIS2_PLACEMENT_3D ( 'NONE', #12241, #32019, #28821 ) ;
#7424=DIRECTION ( 'NONE',  ( 0.000000000000000000, -0.000000000000000000, -1.000000000000000000 ) ) ;
#7445=VERTEX_POINT ( 'NONE', #32570 ) ;
#7467=DIRECTION ( 'NONE',  ( -1.156482317317871232E-16, -0.000000000000000000, -1.000000000000000000 ) ) ;
#7470=AXIS2_PLACEMENT_3D ( 'NONE', #41438, #19515, #31852 ) ;
#7537=CARTESIAN_POINT ( 'NONE',  ( 40.50000000000000711, -7.145751311064596933, 37.00000000000001421 ) ) ;
#7572=DIRECTION ( 'NONE',  ( 0.000000000000000000, -1.000000000000000000, 0.000000000000000000 ) ) ;
#7607=ORIENTED_EDGE ( 'NONE', *, *, #39643, .T. ) ;
#7627=DIRECTION ( 'NONE',  ( -1.000000000000000000, -0.000000000000000000, -0.000000000000000000 ) ) ;
#7646=DIRECTION ( 'NONE',  ( 0.000000000000000000, -1.000000000000000000, 0.000000000000000000 ) ) ;
#7680=CARTESIAN_POINT ( 'NONE',  ( 52.00000000000002132, -2.500000000000000444, -49.99999999999998579 ) ) ;
#7711=CIRCLE ( 'NONE', #30814, 4.000000000000010658 ) ;
#7714=VECTOR ( 'NONE', #37758, 1000.000000000000000 ) ;
#7762=ORIENTED_EDGE ( 'NONE', *, *, #16307, .F. ) ;
#7779=AXIS2_PLACEMENT_3D ( 'NONE', #9306, #38649, #15695 ) ;
#7782=DIRECTION ( 'NONE',  ( 0.000000000000000000, -1.000000000000000000, 0.000000000000000000 ) ) ;
#7819=VERTEX_POINT ( 'NONE', #29331 ) ;
#7831=FACE_OUTER_BOUND ( 'NONE', #42088, .T. ) ;
#7836=AXIS2_PLACEMENT_3D ( 'NONE', #33075, #36485, #19899 ) ;
#7846=LINE ( 'NONE', #14646, #4870 ) ;
#7859=ORIENTED_EDGE ( 'NONE', *, *, #34486, .T. ) ;
#7890=EDGE_CURVE ( 'NONE', #28773, #6804, #38922, .T. ) ;
#7932=CARTESIAN_POINT ( 'NONE',  ( -33.00000000000001421, -4.500000000000000000, 40.00000000000002842 ) ) ;
#7959=ORIENTED_EDGE ( 'NONE', *, *, #20420, .T. ) ;
#7974=ORIENTED_EDGE ( 'NONE', *, *, #2587, .T. ) ;
#7979=ADVANCED_FACE ( 'NONE', ( #21038, #27428 ), #17847, .T. ) ;
#7982=LINE ( 'NONE', #20952, #22094 ) ;
#8011=CARTESIAN_POINT ( 'NONE',  ( 33.00000000000001421, -4.500000000000000000, 40.00000000000002842 ) ) ;
#8162=CARTESIAN_POINT ( 'NONE',  ( 37.52012949071117731, -8.484828722673094958, 40.40326426839882146 ) ) ;
#8175=AXIS2_PLACEMENT_3D ( 'NONE', #31614, #21832, #34805 ) ;
#8190=EDGE_CURVE ( 'NONE', #15408, #40357, #15927, .T. ) ;
#8208=VECTOR ( 'NONE', #19688, 1000.000000000000000 ) ;
#8224=EDGE_CURVE ( 'NONE', #1841, #29490, #20624, .T. ) ;
#8238=VECTOR ( 'NONE', #26040, 1000.000000000000000 ) ;
#8246=CYLINDRICAL_SURFACE ( 'NONE', #34309, 3.000000000000016431 ) ;
#8259=PLANE ( 'NONE',  #24744 ) ;
#8264=EDGE_CURVE ( 'NONE', #6143, #36810, #18685, .T. ) ;
#8276=ADVANCED_FACE ( 'NONE', ( #31648, #22085 ), #5495, .T. ) ;
#8295=DIRECTION ( 'NONE',  ( -0.000000000000000000, -1.000000000000000000, -0.000000000000000000 ) ) ;
#8328=DIRECTION ( 'NONE',  ( 0.000000000000000000, 0.000000000000000000, -1.000000000000000000 ) ) ;
#8350=DIRECTION ( 'NONE',  ( 2.312964634635742957E-16, 1.000000000000000000, 0.000000000000000000 ) ) ;
#8429=ORIENTED_EDGE ( 'NONE', *, *, #29983, .F. ) ;
#8433=ADVANCED_FACE ( 'NONE', ( #41873 ), #32693, .T. ) ;
#8450=DIRECTION ( 'NONE',  ( -1.156482317317871232E-16, 0.000000000000000000, 1.000000000000000000 ) ) ;
#8483=AXIS2_PLACEMENT_3D ( 'NONE', #4007, #33144, #39306 ) ;
#8487=VECTOR ( 'NONE', #7572, 1000.000000000000000 ) ;
#8493=VERTEX_POINT ( 'NONE', #11211 ) ;
#8536=CARTESIAN_POINT ( 'NONE',  ( 11.00000000000000355, 10.00000000000000000, -87.20294101747086302 ) ) ;
#8539=EDGE_LOOP ( 'NONE', ( #3107, #20163, #2836, #39379, #23707, #35005, #8737, #35750 ) ) ;
#8544=EDGE_CURVE ( 'NONE', #31041, #903, #7383, .T. ) ;
#8567=PLANE ( 'NONE',  #2206 ) ;
#8573=CYLINDRICAL_SURFACE ( 'NONE', #28564, 10.00000000000000178 ) ;
#8576=VERTEX_POINT ( 'NONE', #20570 ) ;
#8578=DIRECTION ( 'NONE',  ( 0.000000000000000000, -1.000000000000000000, 0.000000000000000000 ) ) ;
#8600=LINE ( 'NONE', #2431, #18697 ) ;
#8602=DIRECTION ( 'NONE',  ( 0.000000000000000000, 0.000000000000000000, -1.000000000000000000 ) ) ;
#8607=EDGE_CURVE ( 'NONE', #23612, #26597, #23985, .T. ) ;
#8675=DIRECTION ( 'NONE',  ( 0.000000000000000000, 0.000000000000000000, -1.000000000000000000 ) ) ;
#8680=DIRECTION ( 'NONE',  ( -0.000000000000000000, -1.000000000000000000, 0.000000000000000000 ) ) ;
#8685=CARTESIAN_POINT ( 'NONE',  ( 49.99999999999998579, -4.499999999999999112, 44.00000000000002132 ) ) ;
#8689=AXIS2_PLACEMENT_3D ( 'NONE', #39310, #20610, #7424 ) ;
#8723=DIRECTION ( 'NONE',  ( 0.000000000000000000, 1.000000000000000000, 0.000000000000000000 ) ) ;
#8737=ORIENTED_EDGE ( 'NONE', *, *, #7890, .T. ) ;
#8742=DIRECTION ( 'NONE',  ( 0.000000000000000000, 1.000000000000000000, -5.551115123125782702E-16 ) ) ;
#8745=EDGE_CURVE ( 'NONE', #26169, #4135, #34578, .T. ) ;
#8747=CARTESIAN_POINT ( 'NONE',  ( -50.00000000000001421, 10.00000000000000000, 60.00000000000002132 ) ) ;
#8772=DIRECTION ( 'NONE',  ( 0.000000000000000000, -1.000000000000000000, 0.000000000000000000 ) ) ;
#8788=CIRCLE ( 'NONE', #41404, 5.000000000000004441 ) ;
#8828=CARTESIAN_POINT ( 'NONE',  ( -45.00000000000002132, -10.00000000000000000, 60.00000000000002132 ) ) ;
#8845=CIRCLE ( 'NONE', #31244, 4.999999999999997335 ) ;
#8858=LINE ( 'NONE', #18648, #15660 ) ;
#8862=AXIS2_PLACEMENT_3D ( 'NONE', #26263, #10092, #32420 ) ;
#8874=DIRECTION ( 'NONE',  ( 0.000000000000000000, -1.000000000000000000, 0.000000000000000000 ) ) ;
#8880=CARTESIAN_POINT ( 'NONE',  ( -50.00000000000001421, -4.499999999999999112, 44.00000000000003553 ) ) ;
#8897=CARTESIAN_POINT ( 'NONE',  ( -73.31370849898480913, -4.499999999999999112, 44.00000000000003553 ) ) ;
#8911=ORIENTED_EDGE ( 'NONE', *, *, #30364, .F. ) ;
#8933=EDGE_CURVE ( 'NONE', #18435, #5872, #32959, .T. ) ;
#8963=CARTESIAN_POINT ( 'NONE',  ( 49.99999999999998579, -10.00000000000000000, -54.99999999999997158 ) ) ;
#8992=EDGE_LOOP ( 'NONE', ( #3101, #28757, #9913, #30204, #2688 ) ) ;
#9001=VECTOR ( 'NONE', #34845, 1000.000000000000000 ) ;
#9022=EDGE_CURVE ( 'NONE', #8576, #895, #16452, .T. ) ;
#9062=ORIENTED_EDGE ( 'NONE', *, *, #30309, .F. ) ;
#9064=FACE_OUTER_BOUND ( 'NONE', #9382, .T. ) ;
#9073=AXIS2_PLACEMENT_3D ( 'NONE', #16298, #22453, #16100 ) ;
#9082=LINE ( 'NONE', #42055, #26713 ) ;
#9101=CARTESIAN_POINT ( 'NONE',  ( -48.00000000000001421, -10.00000000000000000, 48.35164654424506381 ) ) ;
#9109=VECTOR ( 'NONE', #39076, 1000.000000000000000 ) ;
#9115=FACE_OUTER_BOUND ( 'NONE', #8539, .T. ) ;
#9272=ORIENTED_EDGE ( 'NONE', *, *, #6079, .T. ) ;
#9274=ORIENTED_EDGE ( 'NONE', *, *, #10535, .T. ) ;
#9283=VERTEX_POINT ( 'NONE', #8685 ) ;
#9306=CARTESIAN_POINT ( 'NONE',  ( 49.99999999999998579, -4.500000000000000000, 40.00000000000001421 ) ) ;
#9338=FACE_OUTER_BOUND ( 'NONE', #2045, .T. ) ;
#9376=ORIENTED_EDGE ( 'NONE', *, *, #40363, .F. ) ;
#9381=EDGE_CURVE ( 'NONE', #41347, #12880, #16557, .T. ) ;
#9382=EDGE_LOOP ( 'NONE', ( #28495, #25922, #24051, #3936 ) ) ;
#9403=DIRECTION ( 'NONE',  ( 0.000000000000000000, 0.000000000000000000, -1.000000000000000000 ) ) ;
#9411=CARTESIAN_POINT ( 'NONE',  ( -45.00000000000002132, -2.499999999999999556, -55.00000000000000000 ) ) ;
#9431=VERTEX_POINT ( 'NONE', #29509 ) ;
#9475=ADVANCED_FACE ( 'NONE', ( #3363 ), #29934, .F. ) ;
#9486=ORIENTED_EDGE ( 'NONE', *, *, #18168, .F. ) ;
#9495=EDGE_CURVE ( 'NONE', #15473, #21502, #16349, .T. ) ;
#9522=ORIENTED_EDGE ( 'NONE', *, *, #31551, .F. ) ;
#9546=EDGE_LOOP ( 'NONE', ( #35740, #14405, #4359, #38674, #4617, #34332, #34887, #30141, #32833, #4463, #37990, #11714, #12768, #41140, #34268, #24002 ) ) ;
#9547=CIRCLE ( 'NONE', #8862, 4.999999999999997335 ) ;
#9551=VECTOR ( 'NONE', #8742, 1000.000000000000000 ) ;
#9568=FACE_BOUND ( 'NONE', #38036, .T. ) ;
#9582=LINE ( 'NONE', #10206, #37631 ) ;
#9590=ORIENTED_EDGE ( 'NONE', *, *, #10198, .T. ) ;
#9592=ORIENTED_EDGE ( 'NONE', *, *, #8607, .T. ) ;
#9594=CARTESIAN_POINT ( 'NONE',  ( 47.99999999999998579, 8.000000000000000000, 0.000000000000000000 ) ) ;
#9600=CARTESIAN_POINT ( 'NONE',  ( 62.00000000000002842, -2.499999999999999556, 50.00000000000001421 ) ) ;
#9603=LINE ( 'NONE', #12577, #20709 ) ;
#9655=VECTOR ( 'NONE', #11607, 1000.000000000000000 ) ;
#9683=CARTESIAN_POINT ( 'NONE',  ( 40.50000000000000711, -15.00000000000000000, 40.00000000000002842 ) ) ;
#9696=AXIS2_PLACEMENT_3D ( 'NONE', #3669, #12626, #25605 ) ;
#9706=ORIENTED_EDGE ( 'NONE', *, *, #28198, .F. ) ;
#9711=ORIENTED_EDGE ( 'NONE', *, *, #25999, .F. ) ;
#9718=AXIS2_PLACEMENT_3D ( 'NONE', #18680, #21860, #11864 ) ;
#9781=DIRECTION ( 'NONE',  ( 1.000000000000000000, -0.000000000000000000, 0.000000000000000000 ) ) ;
#9808=AXIS2_PLACEMENT_3D ( 'NONE', #22597, #19604, #9851 ) ;
#9825=EDGE_CURVE ( 'NONE', #746, #33660, #32762, .T. ) ;
#9838=CARTESIAN_POINT ( 'NONE',  ( 40.50000000000000711, 10.00099999999999945, 37.00000000000001421 ) ) ;
#9849=ORIENTED_EDGE ( 'NONE', *, *, #27211, .T. ) ;
#9851=DIRECTION ( 'NONE',  ( 0.000000000000000000, 0.000000000000000000, -1.000000000000000000 ) ) ;
#9852=LINE ( 'NONE', #29383, #41418 ) ;
#9869=AXIS2_PLACEMENT_3D ( 'NONE', #24066, #1906, #37644 ) ;
#9895=CARTESIAN_POINT ( 'NONE',  ( -50.00000000000001421, 10.00000000000000000, -59.99999999999999289 ) ) ;
#9913=ORIENTED_EDGE ( 'NONE', *, *, #25463, .F. ) ;
#9923=ADVANCED_FACE ( 'NONE', ( #1355 ), #8567, .F. ) ;
#9969=VERTEX_POINT ( 'NONE', #31322 ) ;
#9987=DIRECTION ( 'NONE',  ( 0.000000000000000000, -1.000000000000000000, 0.000000000000000000 ) ) ;
#10003=ORIENTED_EDGE ( 'NONE', *, *, #8745, .T. ) ;
#10009=EDGE_CURVE ( 'NONE', #30811, #26169, #18772, .T. ) ;
#10014=DIRECTION ( 'NONE',  ( 0.000000000000000000, 0.000000000000000000, -1.000000000000000000 ) ) ;
#10029=CARTESIAN_POINT ( 'NONE',  ( 40.91258937366526993, -7.170705781850239546, 37.02156881516742004 ) ) ;
#10038=CARTESIAN_POINT ( 'NONE',  ( -50.00000000000001421, 10.00000000000000000, -55.00000000000000000 ) ) ;
#10050=VERTEX_POINT ( 'NONE', #21746 ) ;
#10077=FACE_BOUND ( 'NONE', #23728, .T. ) ;
#10079=CIRCLE ( 'NONE', #35890, 3.000000000000002665 ) ;
#10080=ADVANCED_FACE ( 'NONE', ( #28747 ), #41743, .F. ) ;
#10092=DIRECTION ( 'NONE',  ( -0.000000000000000000, 1.000000000000000000, -0.000000000000000000 ) ) ;
#10120=DIRECTION ( 'NONE',  ( 0.000000000000000000, 0.000000000000000000, 1.000000000000000000 ) ) ;
#10160=DIRECTION ( 'NONE',  ( 0.000000000000000000, 1.000000000000000000, -0.000000000000000000 ) ) ;
#10165=CARTESIAN_POINT ( 'NONE',  ( 44.99999999999999289, -2.499999999999999556, 55.00000000000002132 ) ) ;
#10175=CARTESIAN_POINT ( 'NONE',  ( 9.999999999999998224, 25.00000000000000000, -59.99999999999999289 ) ) ;
#10198=EDGE_CURVE ( 'NONE', #5136, #17804, #32988, .T. ) ;
#10206=CARTESIAN_POINT ( 'NONE',  ( 44.99999999999998579, 10.00000000000000000, -59.99999999999999289 ) ) ;
#10213=VECTOR ( 'NONE', #12042, 1000.000000000000000 ) ;
#10222=ORIENTED_EDGE ( 'NONE', *, *, #18168, .T. ) ;
#10228=EDGE_CURVE ( 'NONE', #27545, #41722, #23431, .T. ) ;
#10238=DIRECTION ( 'NONE',  ( 0.000000000000000000, -1.000000000000000000, 0.000000000000000000 ) ) ;
#10263=EDGE_CURVE ( 'NONE', #4030, #17804, #27390, .T. ) ;
#10295=DIRECTION ( 'NONE',  ( 0.000000000000000000, 0.000000000000000000, 1.000000000000000000 ) ) ;
#10332=MANIFOLD_SOLID_BREP ( 'Boss-Extrude13', #18574 ) ;
#10335=CYLINDRICAL_SURFACE ( 'NONE', #31972, 10.00000000000000178 ) ;
#10352=CARTESIAN_POINT ( 'NONE',  ( -9.999999999999998224, 25.00000000000000000, -87.20294101747086302 ) ) ;
#10399=DIRECTION ( 'NONE',  ( 0.000000000000000000, -1.000000000000000000, 0.000000000000000000 ) ) ;
#10430=DIRECTION ( 'NONE',  ( 0.000000000000000000, 1.000000000000000000, 0.000000000000000000 ) ) ;
#10442=AXIS2_PLACEMENT_3D ( 'NONE', #19552, #3813, #23605 ) ;
#10469=EDGE_LOOP ( 'NONE', ( #3451, #8911, #37070, #9376 ) ) ;
#10470=DIRECTION ( 'NONE',  ( 1.000000000000000000, 0.000000000000000000, 0.000000000000000000 ) ) ;
#10516=CARTESIAN_POINT ( 'NONE',  ( 37.81994042647383480, -8.265607769982835862, 41.36257643287451913 ) ) ;
#10535=EDGE_CURVE ( 'NONE', #25761, #35430, #25528, .T. ) ;
#10539=ORIENTED_EDGE ( 'NONE', *, *, #25644, .T. ) ;
#10566=LINE ( 'NONE', #17576, #21069 ) ;
#10577=AXIS2_PLACEMENT_3D ( 'NONE', #18347, #8772, #2180 ) ;
#10579=DIRECTION ( 'NONE',  ( 0.000000000000000000, 0.000000000000000000, -1.000000000000000000 ) ) ;
#10612=PLANE ( 'NONE',  #19998 ) ;
#10659=CARTESIAN_POINT ( 'NONE',  ( 43.08079448876115691, -8.195172673408354314, 41.54134514533654965 ) ) ;
#10731=ORIENTED_EDGE ( 'NONE', *, *, #5879, .F. ) ;
#10742=ORIENTED_EDGE ( 'NONE', *, *, #13148, .T. ) ;
#10756=DIRECTION ( 'NONE',  ( 0.000000000000000000, -1.000000000000000000, 0.000000000000000000 ) ) ;
#10767=DIRECTION ( 'NONE',  ( 0.000000000000000000, 1.000000000000000000, -0.000000000000000000 ) ) ;
#10797=CARTESIAN_POINT ( 'NONE',  ( 47.99999999999998579, -4.500000000000000888, 50.00000000000002842 ) ) ;
#10813=CARTESIAN_POINT ( 'NONE',  ( 11.00000000000000355, 10.00000000000000000, -59.99999999999999289 ) ) ;
#10828=VECTOR ( 'NONE', #27339, 1000.000000000000000 ) ;
#10839=ORIENTED_EDGE ( 'NONE', *, *, #11044, .F. ) ;
#10847=VECTOR ( 'NONE', #5072, 1000.000000000000000 ) ;
#10850=LINE ( 'NONE', #23837, #6308 ) ;
#10867=CARTESIAN_POINT ( 'NONE',  ( 42.86524676284565771, -8.047984377394540090, 41.85522311356901071 ) ) ;
#10868=CARTESIAN_POINT ( 'NONE',  ( 62.00000000000001421, 2.499999999999999556, -60.00000000000000000 ) ) ;
#10878=( LENGTH_UNIT ( ) NAMED_UNIT ( * ) SI_UNIT ( .MILLI., .METRE. ) );
#10893=PRODUCT_DEFINITION_SHAPE ( 'NONE', 'NONE',  #22866 ) ;
#10896=EDGE_LOOP ( 'NONE', ( #38931, #7195, #24558, #20142, #2161, #31457 ) ) ;
#10899=ORIENTED_EDGE ( 'NONE', *, *, #31681, .F. ) ;
#10906=CARTESIAN_POINT ( 'NONE',  ( -33.00000000000001421, -4.500000000000000000, 40.00000000000002842 ) ) ;
#10916=( NAMED_UNIT ( * ) SI_UNIT ( $, .STERADIAN. ) SOLID_ANGLE_UNIT ( ) );
#10920=EDGE_CURVE ( 'NONE', #4822, #18848, #1265, .T. ) ;
#10938=CARTESIAN_POINT ( 'NONE',  ( -9.999999999999998224, 25.00000000000000000, -87.20294101747086302 ) ) ;
#11023=AXIS2_PLACEMENT_3D ( 'NONE', #18060, #11260, #17852 ) ;
#11030=CARTESIAN_POINT ( 'NONE',  ( -33.00000000000001421, 7.999999999999996447, 50.00000000000002842 ) ) ;
#11042=FACE_OUTER_BOUND ( 'NONE', #9546, .T. ) ;
#11044=EDGE_CURVE ( 'NONE', #14857, #22137, #36199, .T. ) ;
#11054=CARTESIAN_POINT ( 'NONE',  ( 40.50000000000000711, -15.00000000000000000, 36.00000000000002132 ) ) ;
#11056=VECTOR ( 'NONE', #9403, 1000.000000000000000 ) ;
#11057=VERTEX_POINT ( 'NONE', #31850 ) ;
#11083=VECTOR ( 'NONE', #5722, 1000.000000000000000 ) ;
#11112=DIRECTION ( 'NONE',  ( 0.000000000000000000, 0.000000000000000000, 1.000000000000000000 ) ) ;
#11117=EDGE_LOOP ( 'NONE', ( #28407, #28464, #15409, #32161 ) ) ;
#11118=LINE ( 'NONE', #36639, #910 ) ;
#11131=CARTESIAN_POINT ( 'NONE',  ( 0.000000000000000000, 0.000000000000000000, 0.000000000000000000 ) ) ;
#11161=DIRECTION ( 'NONE',  ( 0.000000000000000000, 0.000000000000000000, 1.000000000000000000 ) ) ;
#11170=CARTESIAN_POINT ( 'NONE',  ( 10.00000000000000178, 10.00000000000000000, 60.00000000000002132 ) ) ;
#11176=CARTESIAN_POINT ( 'NONE',  ( -45.00000000000002132, 10.00000000000000000, 55.00000000000002132 ) ) ;
#11178=VECTOR ( 'NONE', #35143, 1000.000000000000000 ) ;
#11181=CARTESIAN_POINT ( 'NONE',  ( 40.50000000000000711, -10.00000000000000000, 40.00000000000002842 ) ) ;
#11211=CARTESIAN_POINT ( 'NONE',  ( 49.99999999999998579, 2.499999999999999556, 55.00000000000002132 ) ) ;
#11226=ORIENTED_EDGE ( 'NONE', *, *, #17113, .T. ) ;
#11260=DIRECTION ( 'NONE',  ( 1.000000000000000000, 0.000000000000000000, 0.000000000000000000 ) ) ;
#11262=ORIENTED_EDGE ( 'NONE', *, *, #37280, .T. ) ;
#11268=EDGE_CURVE ( 'NONE', #40357, #41076, #32795, .T. ) ;
#11314=ORIENTED_EDGE ( 'NONE', *, *, #16347, .F. ) ;
#11316=CYLINDRICAL_SURFACE ( 'NONE', #30786, 10.00000000000000178 ) ;
#11338=CARTESIAN_POINT ( 'NONE',  ( -52.00000000000002842, 2.499999999999999556, 50.00000000000001421 ) ) ;
#11367=LINE ( 'NONE', #23514, #19874 ) ;
#11391=EDGE_CURVE ( 'NONE', #11983, #40855, #9082, .T. ) ;
#11456=ORIENTED_EDGE ( 'NONE', *, *, #18544, .F. ) ;
#11497=CARTESIAN_POINT ( 'NONE',  ( -62.00000000000002842, 2.499999999999999556, 50.00000000000001421 ) ) ;
#11508=LINE ( 'NONE', #40241, #12293 ) ;
#11515=ORIENTED_EDGE ( 'NONE', *, *, #4634, .T. ) ;
#11523=ORIENTED_EDGE ( 'NONE', *, *, #3118, .T. ) ;
#11527=VECTOR ( 'NONE', #28659, 1000.000000000000000 ) ;
#11535=CARTESIAN_POINT ( 'NONE',  ( -48.00000000000001421, 8.000000000000000000, 30.00000000000002132 ) ) ;
#11560=ORIENTED_EDGE ( 'NONE', *, *, #2587, .F. ) ;
#11570=ORIENTED_EDGE ( 'NONE', *, *, #9022, .F. ) ;
#11583=VECTOR ( 'NONE', #5060, 1000.000000000000000 ) ;
#11607=DIRECTION ( 'NONE',  ( 1.000000000000000000, -0.000000000000000000, -0.000000000000000000 ) ) ;
#11673=ORIENTED_EDGE ( 'NONE', *, *, #15480, .T. ) ;
#11706=ORIENTED_EDGE ( 'NONE', *, *, #39460, .T. ) ;
#11714=ORIENTED_EDGE ( 'NONE', *, *, #6965, .T. ) ;
#11728=MECHANICAL_DESIGN_GEOMETRIC_PRESENTATION_REPRESENTATION('',(#41660),#4936);
#11729=DIRECTION ( 'NONE',  ( -1.000000000000000000, 0.000000000000000000, 0.000000000000000000 ) ) ;
#11761=LINE ( 'NONE', #14965, #22976 ) ;
#11764=CARTESIAN_POINT ( 'NONE',  ( -52.00000000000001421, -2.499999999999999556, -60.00000000000000000 ) ) ;
#11782=LINE ( 'NONE', #17761, #20715 ) ;
#11786=EDGE_CURVE ( 'NONE', #38231, #37461, #13525, .T. ) ;
#11818=EDGE_CURVE ( 'NONE', #16482, #15473, #12010, .T. ) ;
#11833=DIRECTION ( 'NONE',  ( 0.000000000000000000, -1.734723475976806108E-16, 1.000000000000000000 ) ) ;
#11834=AXIS2_PLACEMENT_3D ( 'NONE', #29222, #13287, #13077 ) ;
#11836=DIRECTION ( 'NONE',  ( 0.000000000000000000, -1.000000000000000000, -0.000000000000000000 ) ) ;
#11864=DIRECTION ( 'NONE',  ( 0.000000000000000000, 0.000000000000000000, -1.000000000000000000 ) ) ;
#11867=CARTESIAN_POINT ( 'NONE',  ( -50.00000000000001421, 2.499999999999999556, -55.00000000000000000 ) ) ;
#11873=EDGE_CURVE ( 'NONE', #8576, #1429, #30534, .T. ) ;
#11912=CARTESIAN_POINT ( 'NONE',  ( 48.00000000000001421, -4.500000000000000000, 40.00000000000002842 ) ) ;
#11921=CIRCLE ( 'NONE', #10577, 4.000000000000010658 ) ;
#11936=DIRECTION ( 'NONE',  ( 1.000000000000000000, 0.000000000000000000, 0.000000000000000000 ) ) ;
#11941=CARTESIAN_POINT ( 'NONE',  ( 33.00000000000001421, -4.499999999999999112, 44.00000000000003553 ) ) ;
#11944=ORIENTED_EDGE ( 'NONE', *, *, #33184, .T. ) ;
#11969=FACE_OUTER_BOUND ( 'NONE', #26755, .T. ) ;
#11970=DIRECTION ( 'NONE',  ( 0.000000000000000000, 0.000000000000000000, -1.000000000000000000 ) ) ;
#11974=CARTESIAN_POINT ( 'NONE',  ( 0.000000000000000000, 10.00000000000000000, 0.000000000000000000 ) ) ;
#11983=VERTEX_POINT ( 'NONE', #18613 ) ;
#12010=LINE ( 'NONE', #4591, #37581 ) ;
#12028=CARTESIAN_POINT ( 'NONE',  ( 33.00000000000001421, 8.000000000000000000, 30.00000000000002132 ) ) ;
#12042=DIRECTION ( 'NONE',  ( 0.000000000000000000, 1.000000000000000000, -5.551115123125782702E-16 ) ) ;
#12064=DIRECTION ( 'NONE',  ( 1.000000000000000000, -0.000000000000000000, -1.067522139062650178E-16 ) ) ;
#12072=LINE ( 'NONE', #5281, #10847 ) ;
#12181=VECTOR ( 'NONE', #26978, 1000.000000000000000 ) ;
#12198=VECTOR ( 'NONE', #6733, 1000.000000000000000 ) ;
#12235=EDGE_CURVE ( 'NONE', #8576, #23938, #20287, .T. ) ;
#12236=DIRECTION ( 'NONE',  ( 0.000000000000000000, 0.000000000000000000, 1.000000000000000000 ) ) ;
#12241=CARTESIAN_POINT ( 'NONE',  ( 44.99999999999998579, 8.000000000000000000, -54.99999999999999289 ) ) ;
#12243=ORIENTED_EDGE ( 'NONE', *, *, #11818, .T. ) ;
#12244=ORIENTED_EDGE ( 'NONE', *, *, #3630, .T. ) ;
#12254=LINE ( 'NONE', #19061, #38046 ) ;
#12269=CARTESIAN_POINT ( 'NONE',  ( 40.50000000000000711, -10.00000000000000000, 44.00000000000004263 ) ) ;
#12276=DIRECTION ( 'NONE',  ( 0.000000000000000000, 0.000000000000000000, -1.000000000000000000 ) ) ;
#12279=CYLINDRICAL_SURFACE ( 'NONE', #36371, 4.000000000000003553 ) ;
#12293=VECTOR ( 'NONE', #11112, 1000.000000000000000 ) ;
#12294=CARTESIAN_POINT ( 'NONE',  ( -62.00000000000002842, -2.499999999999999556, 36.53589838486226427 ) ) ;
#12351=EDGE_LOOP ( 'NONE', ( #107, #17611, #15613, #40508, #35426, #2662 ) ) ;
#12359=CARTESIAN_POINT ( 'NONE',  ( 62.00000000000002842, -2.499999999999999556, 60.00000000000002132 ) ) ;
#12362=CARTESIAN_POINT ( 'NONE',  ( 49.99999999999998579, -2.499999999999999556, 55.00000000000002132 ) ) ;
#12364=CARTESIAN_POINT ( 'NONE',  ( -73.31370849898480913, -4.500000000000000000, 40.00000000000002842 ) ) ;
#12375=AXIS2_PLACEMENT_3D ( 'NONE', #28335, #25580, #38541 ) ;
#12398=DIRECTION ( 'NONE',  ( -0.000000000000000000, 1.000000000000000000, -0.000000000000000000 ) ) ;
#12455=EDGE_CURVE ( 'NONE', #31393, #37469, #28674, .T. ) ;
#12504=APPLICATION_CONTEXT ( 'automotive_design' ) ;
#12521=ORIENTED_EDGE ( 'NONE', *, *, #4888, .F. ) ;
#12555=AXIS2_PLACEMENT_3D ( 'NONE', #7680, #8295, #24889 ) ;
#12567=DIRECTION ( 'NONE',  ( 0.000000000000000000, 0.000000000000000000, -1.000000000000000000 ) ) ;
#12576=ORIENTED_EDGE ( 'NONE', *, *, #36365, .T. ) ;
#12577=CARTESIAN_POINT ( 'NONE',  ( 0.000000000000000000, -10.00000000000000000, 58.00000000000001421 ) ) ;
#12582=CIRCLE ( 'NONE', #7836, 10.00000000000000178 ) ;
#12599=VECTOR ( 'NONE', #33796, 1000.000000000000000 ) ;
#12609=VERTEX_POINT ( 'NONE', #33806 ) ;
#12626=DIRECTION ( 'NONE',  ( -0.000000000000000000, -1.000000000000000000, 0.000000000000000000 ) ) ;
#12646=LINE ( 'NONE', #25626, #25311 ) ;
#12659=CARTESIAN_POINT ( 'NONE',  ( -50.00000000000001421, -10.00000000000000000, -54.99999999999997158 ) ) ;
#12663=ORIENTED_EDGE ( 'NONE', *, *, #1945, .F. ) ;
#12681=DIRECTION ( 'NONE',  ( -0.000000000000000000, -1.000000000000000000, -0.000000000000000000 ) ) ;
#12687=CARTESIAN_POINT ( 'NONE',  ( 49.99999999999998579, -4.500000000000000000, 40.00000000000001421 ) ) ;
#12724=DIRECTION ( 'NONE',  ( 1.000000000000000000, -0.000000000000000000, 0.000000000000000000 ) ) ;
#12726=CARTESIAN_POINT ( 'NONE',  ( 44.99999999999999289, 10.00000000000000000, 55.00000000000002132 ) ) ;
#12729=CARTESIAN_POINT ( 'NONE',  ( 40.50000000000000711, -7.145751311064596933, 37.00000000000001421 ) ) ;
#12768=ORIENTED_EDGE ( 'NONE', *, *, #4725, .T. ) ;
#12828=EDGE_CURVE ( 'NONE', #5136, #16152, #24291, .T. ) ;
#12838=CARTESIAN_POINT ( 'NONE',  ( 48.00000000000001421, -4.500000000000000000, 40.00000000000002842 ) ) ;
#12840=AXIS2_PLACEMENT_3D ( 'NONE', #34115, #14562, #11161 ) ;
#12880=VERTEX_POINT ( 'NONE', #40905 ) ;
#12915=FACE_OUTER_BOUND ( 'NONE', #25444, .T. ) ;
#12922=ORIENTED_EDGE ( 'NONE', *, *, #15282, .T. ) ;
#12946=ADVANCED_FACE ( 'NONE', ( #41335 ), #31128, .F. ) ;
#12962=AXIS2_PLACEMENT_3D ( 'NONE', #24811, #31593, #28191 ) ;
#12980=ORIENTED_EDGE ( 'NONE', *, *, #16861, .T. ) ;
#12985=ORIENTED_EDGE ( 'NONE', *, *, #6159, .F. ) ;
#13040=VERTEX_POINT ( 'NONE', #28972 ) ;
#13077=DIRECTION ( 'NONE',  ( 0.000000000000000000, -0.000000000000000000, -1.000000000000000000 ) ) ;
#13092=CARTESIAN_POINT ( 'NONE',  ( -73.31370849898480913, -2.499999999999999556, 36.53589838486226427 ) ) ;
#13108=VECTOR ( 'NONE', #18122, 1000.000000000000000 ) ;
#13122=PLANE ( 'NONE',  #13599 ) ;
#13128=ORIENTED_EDGE ( 'NONE', *, *, #11268, .F. ) ;
#13146=EDGE_LOOP ( 'NONE', ( #40305, #3308, #21254, #41446, #24402, #39913 ) ) ;
#13148=EDGE_CURVE ( 'NONE', #33660, #37461, #680, .T. ) ;
#13150=EDGE_CURVE ( 'NONE', #9969, #28880, #4217, .T. ) ;
#13169=PLANE ( 'NONE',  #1240 ) ;
#13177=CARTESIAN_POINT ( 'NONE',  ( 47.99999999999998579, 10.00000000000000000, -54.99999999999997158 ) ) ;
#13199=VERTEX_POINT ( 'NONE', #8828 ) ;
#13206=VERTEX_POINT ( 'NONE', #18617 ) ;
#13212=EDGE_CURVE ( 'NONE', #26584, #6074, #37550, .T. ) ;
#13213=CARTESIAN_POINT ( 'NONE',  ( 42.47658145770895999, -7.800883640287679555, 37.73528810251997356 ) ) ;
#13220=CIRCLE ( 'NONE', #12555, 10.00000000000000178 ) ;
#13287=DIRECTION ( 'NONE',  ( 0.000000000000000000, -1.000000000000000000, 0.000000000000000000 ) ) ;
#13307=VECTOR ( 'NONE', #10756, 1000.000000000000000 ) ;
#13316=EDGE_CURVE ( 'NONE', #10050, #20613, #31581, .T. ) ;
#13332=ADVANCED_FACE ( 'NONE', ( #27765 ), #34361, .T. ) ;
#13344=CARTESIAN_POINT ( 'NONE',  ( -45.00000000000002132, 10.00000000000000000, -59.99999999999999289 ) ) ;
#13352=VERTEX_POINT ( 'NONE', #24586 ) ;
#13402=ADVANCED_FACE ( 'NONE', ( #5006 ), #21589, .T. ) ;
#13414=CARTESIAN_POINT ( 'NONE',  ( 40.70723611629013305, -7.145751311064572953, 43.00000000000004974 ) ) ;
#13438=EDGE_LOOP ( 'NONE', ( #19566, #25119, #864, #34806 ) ) ;
#13444=ORIENTED_EDGE ( 'NONE', *, *, #14132, .F. ) ;
#13449=ORIENTED_EDGE ( 'NONE', *, *, #17092, .F. ) ;
#13459=CARTESIAN_POINT ( 'NONE',  ( 48.00000000000001421, 7.999999999999996447, 50.00000000000002842 ) ) ;
#13465=DIRECTION ( 'NONE',  ( -0.000000000000000000, -1.000000000000000000, 0.000000000000000000 ) ) ;
#13479=DIRECTION ( 'NONE',  ( 0.000000000000000000, 0.000000000000000000, 1.000000000000000000 ) ) ;
#13516=CARTESIAN_POINT ( 'NONE',  ( -48.00000000000001421, 8.000000000000000000, 0.000000000000000000 ) ) ;
#13525=LINE ( 'NONE', #39471, #31463 ) ;
#13579=DIRECTION ( 'NONE',  ( 0.000000000000000000, -1.000000000000000000, 0.000000000000000000 ) ) ;
#13599=AXIS2_PLACEMENT_3D ( 'NONE', #26104, #39062, #29482 ) ;
#13602=DIRECTION ( 'NONE',  ( -1.000000000000000000, 0.000000000000000000, -1.156482317317871232E-16 ) ) ;
#13611=FACE_OUTER_BOUND ( 'NONE', #32139, .T. ) ;
#13621=AXIS2_PLACEMENT_3D ( 'NONE', #16544, #29279, #32688 ) ;
#13639=DIRECTION ( 'NONE',  ( -0.000000000000000000, 5.551115123125782702E-16, 1.000000000000000000 ) ) ;
#13654=DIRECTION ( 'NONE',  ( 0.000000000000000000, 0.000000000000000000, -1.000000000000000000 ) ) ;
#13659=VECTOR ( 'NONE', #21022, 1000.000000000000000 ) ;
#13667=ADVANCED_FACE ( 'NONE', ( #33338 ), #33972, .F. ) ;
#13700=VECTOR ( 'NONE', #7467, 1000.000000000000000 ) ;
#13703=CARTESIAN_POINT ( 'NONE',  ( 37.82603108925543012, -8.261268920114268610, 38.62561309397396769 ) ) ;
#13714=ORIENTED_EDGE ( 'NONE', *, *, #13942, .F. ) ;
#13718=AXIS2_PLACEMENT_3D ( 'NONE', #36134, #7646, #33373 ) ;
#13744=DIRECTION ( 'NONE',  ( 0.000000000000000000, -1.000000000000000000, 0.000000000000000000 ) ) ;
#13754=DIRECTION ( 'NONE',  ( 0.000000000000000000, 0.000000000000000000, -1.000000000000000000 ) ) ;
#13771=CARTESIAN_POINT ( 'NONE',  ( 47.99999999999998579, 8.000000000000000000, 0.000000000000000000 ) ) ;
#13778=CARTESIAN_POINT ( 'NONE',  ( -11.00000000000000355, 26.00000000000000355, 60.00000000000002132 ) ) ;
#13780=VERTEX_POINT ( 'NONE', #10797 ) ;
#13784=EDGE_CURVE ( 'NONE', #38216, #36810, #29339, .T. ) ;
#13831=DIRECTION ( 'NONE',  ( 1.000000000000000000, 0.000000000000000000, 0.000000000000000000 ) ) ;
#13836=ORIENTED_EDGE ( 'NONE', *, *, #26453, .F. ) ;
#13840=CIRCLE ( 'NONE', #35582, 4.999999999999997335 ) ;
#13844=CARTESIAN_POINT ( 'NONE',  ( 42.33205937540029851, -7.715456146116813407, 37.61698112454933352 ) ) ;
#13853=CARTESIAN_POINT ( 'NONE',  ( 44.99999999999998579, 10.00000000000000000, 60.00000000000002132 ) ) ;
#13875=FACE_OUTER_BOUND ( 'NONE', #13438, .T. ) ;
#13908=CARTESIAN_POINT ( 'NONE',  ( 48.00000000000001421, -4.500000000000000000, 30.00000000000002842 ) ) ;
#13915=CARTESIAN_POINT ( 'NONE',  ( 37.91570509911780817, -8.197609404464536453, 41.53566612860994667 ) ) ;
#13942=EDGE_CURVE ( 'NONE', #16152, #4030, #35219, .T. ) ;
#13945=ADVANCED_FACE ( 'NONE', ( #2894 ), #2475, .T. ) ;
#13959=LINE ( 'NONE', #1404, #41578 ) ;
#13975=CIRCLE ( 'NONE', #35704, 3.000000000000002665 ) ;
#13987=ORIENTED_EDGE ( 'NONE', *, *, #36416, .F. ) ;
#14004=CARTESIAN_POINT ( 'NONE',  ( 40.50000000000000711, -15.00000000000000000, 44.00000000000004263 ) ) ;
#14005=ADVANCED_FACE ( 'NONE', ( #9064 ), #31811, .T. ) ;
#14006=VECTOR ( 'NONE', #31505, 1000.000000000000000 ) ;
#14087=CARTESIAN_POINT ( 'NONE',  ( 62.00000000000002842, 2.499999999999999556, 50.00000000000001421 ) ) ;
#14127=DIRECTION ( 'NONE',  ( 0.000000000000000000, -1.000000000000000000, 0.000000000000000000 ) ) ;
#14132=EDGE_CURVE ( 'NONE', #31292, #37304, #40979, .T. ) ;
#14185=LINE ( 'NONE', #27162, #6260 ) ;
#14201=DIRECTION ( 'NONE',  ( 1.156482317317871232E-16, 0.000000000000000000, -1.000000000000000000 ) ) ;
#14216=DIRECTION ( 'NONE',  ( -0.000000000000000000, -1.000000000000000000, -0.000000000000000000 ) ) ;
#14267=ADVANCED_FACE ( 'NONE', ( #29039 ), #32853, .T. ) ;
#14339=ORIENTED_EDGE ( 'NONE', *, *, #20955, .T. ) ;
#14342=CARTESIAN_POINT ( 'NONE',  ( 39.14897100094481885, -7.466300162885855407, 42.68550559702568137 ) ) ;
#14350=ORIENTED_EDGE ( 'NONE', *, *, #34025, .T. ) ;
#14398=DIRECTION ( 'NONE',  ( -0.000000000000000000, -0.000000000000000000, 1.000000000000000000 ) ) ;
#14401=ORIENTED_EDGE ( 'NONE', *, *, #21193, .F. ) ;
#14405=ORIENTED_EDGE ( 'NONE', *, *, #37253, .T. ) ;
#14414=LINE ( 'NONE', #24000, #23795 ) ;
#14415=ORIENTED_EDGE ( 'NONE', *, *, #29406, .F. ) ;
#14443=DIRECTION ( 'NONE',  ( 0.000000000000000000, 0.000000000000000000, 1.000000000000000000 ) ) ;
#14453=ADVANCED_FACE ( 'NONE', ( #39660 ), #36476, .F. ) ;
#14472=EDGE_CURVE ( 'NONE', #1211, #16482, #11367, .T. ) ;
#14483=AXIS2_PLACEMENT_3D ( 'NONE', #16194, #29345, #10014 ) ;
#14520=VERTEX_POINT ( 'NONE', #21567 ) ;
#14562=DIRECTION ( 'NONE',  ( -1.000000000000000000, 0.000000000000000000, 0.000000000000000000 ) ) ;
#14564=ORIENTED_EDGE ( 'NONE', *, *, #31287, .F. ) ;
#14583=DIRECTION ( 'NONE',  ( 0.000000000000000000, 0.000000000000000000, -1.000000000000000000 ) ) ;
#14646=CARTESIAN_POINT ( 'NONE',  ( -62.00000000000001421, 2.499999999999999556, -49.99999999999998579 ) ) ;
#14657=CARTESIAN_POINT ( 'NONE',  ( -33.00000000000001421, -4.500000000000000000, 30.00000000000002842 ) ) ;
#14681=ORIENTED_EDGE ( 'NONE', *, *, #30067, .T. ) ;
#14734=CARTESIAN_POINT ( 'NONE',  ( 49.99999999999998579, -4.500000000000000000, 36.00000000000001421 ) ) ;
#14749=EDGE_CURVE ( 'NONE', #25504, #15972, #22578, .T. ) ;
#14771=EDGE_CURVE ( 'NONE', #37769, #37304, #20556, .T. ) ;
#14773=EDGE_LOOP ( 'NONE', ( #13444, #22237, #5277, #38412, #31185, #5869 ) ) ;
#14788=DIRECTION ( 'NONE',  ( 0.000000000000000000, 0.000000000000000000, -1.000000000000000000 ) ) ;
#14800=CARTESIAN_POINT ( 'NONE',  ( -50.00000000000001421, 10.00000000000000000, 60.00000000000002132 ) ) ;
#14857=VERTEX_POINT ( 'NONE', #3884 ) ;
#14880=ORIENTED_EDGE ( 'NONE', *, *, #11044, .T. ) ;
#14891=DIRECTION ( 'NONE',  ( 0.000000000000000000, 0.000000000000000000, 1.000000000000000000 ) ) ;
#14898=DIRECTION ( 'NONE',  ( 0.000000000000000000, 0.000000000000000000, -1.000000000000000000 ) ) ;
#14911=ORIENTED_EDGE ( 'NONE', *, *, #646, .F. ) ;
#14920=VECTOR ( 'NONE', #7084, 1000.000000000000000 ) ;
#14921=ADVANCED_FACE ( 'NONE', ( #40462 ), #11316, .T. ) ;
#14944=EDGE_CURVE ( 'NONE', #39331, #15473, #11118, .T. ) ;
#14965=CARTESIAN_POINT ( 'NONE',  ( -62.00000000000002842, 2.499999999999999556, 50.00000000000001421 ) ) ;
#14980=ORIENTED_EDGE ( 'NONE', *, *, #33232, .F. ) ;
#14987=DIRECTION ( 'NONE',  ( 0.000000000000000000, -1.000000000000000000, 0.000000000000000000 ) ) ;
#15039=EDGE_CURVE ( 'NONE', #7445, #37476, #41294, .T. ) ;
#15049=ORIENTED_EDGE ( 'NONE', *, *, #33184, .F. ) ;
#15053=FACE_BOUND ( 'NONE', #41768, .T. ) ;
#15054=DIRECTION ( 'NONE',  ( 0.000000000000000000, -1.000000000000000000, 0.000000000000000000 ) ) ;
#15060=DIRECTION ( 'NONE',  ( -0.000000000000000000, 1.000000000000000000, -0.000000000000000000 ) ) ;
#15082=EDGE_LOOP ( 'NONE', ( #34639, #32740, #15256, #26068 ) ) ;
#15084=DIRECTION ( 'NONE',  ( 0.000000000000000000, 1.000000000000000000, 0.000000000000000000 ) ) ;
#15085=VECTOR ( 'NONE', #798, 1000.000000000000000 ) ;
#15089=CARTESIAN_POINT ( 'NONE',  ( -50.00000000000001421, 10.00000000000000000, 60.00000000000002132 ) ) ;
#15093=EDGE_CURVE ( 'NONE', #41722, #40514, #40659, .T. ) ;
#15103=CARTESIAN_POINT ( 'NONE',  ( -45.00000000000002132, 8.000000000000000000, -55.00000000000000000 ) ) ;
#15138=ORIENTED_EDGE ( 'NONE', *, *, #40890, .T. ) ;
#15174=CARTESIAN_POINT ( 'NONE',  ( 33.00000000000001421, 8.000000000000000000, 30.00000000000002132 ) ) ;
#15181=VECTOR ( 'NONE', #32530, 1000.000000000000000 ) ;
#15200=AXIS2_PLACEMENT_3D ( 'NONE', #15699, #34833, #31638 ) ;
#15214=CARTESIAN_POINT ( 'NONE',  ( -33.00000000000001421, -10.00000000000000000, 31.64835345575499304 ) ) ;
#15255=AXIS2_PLACEMENT_3D ( 'NONE', #36242, #7114, #6691 ) ;
#15256=ORIENTED_EDGE ( 'NONE', *, *, #40942, .F. ) ;
#15277=EDGE_LOOP ( 'NONE', ( #31757, #24612, #7762, #23357 ) ) ;
#15282=EDGE_CURVE ( 'NONE', #3926, #5504, #22610, .T. ) ;
#15288=FACE_OUTER_BOUND ( 'NONE', #19475, .T. ) ;
#15302=ADVANCED_FACE ( 'NONE', ( #19163 ), #35746, .T. ) ;
#15338=DIRECTION ( 'NONE',  ( 1.000000000000000000, -0.000000000000000000, -0.000000000000000000 ) ) ;
#15357=CARTESIAN_POINT ( 'NONE',  ( 11.00000000000000355, 26.00000000000000355, -59.99999999999999289 ) ) ;
#15408=VERTEX_POINT ( 'NONE', #22975 ) ;
#15409=ORIENTED_EDGE ( 'NONE', *, *, #22155, .T. ) ;
#15414=CARTESIAN_POINT ( 'NONE',  ( 44.99999999999998579, -10.00000000000000000, -59.99999999999999289 ) ) ;
#15416=FACE_OUTER_BOUND ( 'NONE', #15277, .T. ) ;
#15425=CARTESIAN_POINT ( 'NONE',  ( 44.99999999999999289, -2.499999999999999556, 55.00000000000002132 ) ) ;
#15457=ORIENTED_EDGE ( 'NONE', *, *, #19160, .T. ) ;
#15473=VERTEX_POINT ( 'NONE', #1487 ) ;
#15478=DIRECTION ( 'NONE',  ( 0.000000000000000000, 0.000000000000000000, -1.000000000000000000 ) ) ;
#15480=EDGE_CURVE ( 'NONE', #35430, #16352, #27022, .T. ) ;
#15501=CARTESIAN_POINT ( 'NONE',  ( 44.99999999999998579, 10.00000000000000000, -59.99999999999999289 ) ) ;
#15512=EDGE_CURVE ( 'NONE', #3104, #29446, #10850, .T. ) ;
#15530=ADVANCED_FACE ( 'NONE', ( #13611 ), #39985, .T. ) ;
#15553=ORIENTED_EDGE ( 'NONE', *, *, #16307, .T. ) ;
#15564=FACE_OUTER_BOUND ( 'NONE', #38283, .T. ) ;
#15605=PLANE ( 'NONE',  #2637 ) ;
#15613=ORIENTED_EDGE ( 'NONE', *, *, #5050, .F. ) ;
#15628=DIRECTION ( 'NONE',  ( 0.000000000000000000, -1.000000000000000000, 0.000000000000000000 ) ) ;
#15630=EDGE_CURVE ( 'NONE', #37304, #39773, #30621, .T. ) ;
#15660=VECTOR ( 'NONE', #11833, 1000.000000000000000 ) ;
#15695=DIRECTION ( 'NONE',  ( 0.000000000000000000, 0.000000000000000000, 1.000000000000000000 ) ) ;
#15699=CARTESIAN_POINT ( 'NONE',  ( 49.99999999999998579, -4.500000000000000000, 40.00000000000001421 ) ) ;
#15705=CARTESIAN_POINT ( 'NONE',  ( -44.99999999999998579, -2.499999999999999556, -60.00000000000000000 ) ) ;
#15709=CARTESIAN_POINT ( 'NONE',  ( -33.00000000000001421, -4.500000000000000000, 40.00000000000002842 ) ) ;
#15719=PLANE ( 'NONE',  #23537 ) ;
#15723=EDGE_CURVE ( 'NONE', #39331, #38083, #31040, .T. ) ;
#15740=AXIS2_PLACEMENT_3D ( 'NONE', #2069, #15054, #15478 ) ;
#15763=ORIENTED_EDGE ( 'NONE', *, *, #22629, .T. ) ;
#15812=EDGE_CURVE ( 'NONE', #8493, #28773, #34849, .T. ) ;
#15826=AXIS2_PLACEMENT_3D ( 'NONE', #27453, #4895, #27649 ) ;
#15827=CARTESIAN_POINT ( 'NONE',  ( -48.00000000000001421, 8.000000000000000000, 0.000000000000000000 ) ) ;
#15880=ORIENTED_EDGE ( 'NONE', *, *, #34025, .F. ) ;
#15889=AXIS2_PLACEMENT_3D ( 'NONE', #28553, #41751, #3239 ) ;
#15910=CARTESIAN_POINT ( 'NONE',  ( 44.99999999999998579, 10.00000000000000000, -54.99999999999999289 ) ) ;
#15927=LINE ( 'NONE', #15501, #31385 ) ;
#15972=VERTEX_POINT ( 'NONE', #39093 ) ;
#15982=ORIENTED_EDGE ( 'NONE', *, *, #21049, .F. ) ;
#16011=DIRECTION ( 'NONE',  ( 0.000000000000000000, -1.000000000000000000, 0.000000000000000000 ) ) ;
#16016=DIRECTION ( 'NONE',  ( 0.000000000000000000, 1.000000000000000000, -5.551115123125782702E-16 ) ) ;
#16029=EDGE_CURVE ( 'NONE', #6615, #1179, #32709, .T. ) ;
#16039=VERTEX_POINT ( 'NONE', #3572 ) ;
#16042=ORIENTED_EDGE ( 'NONE', *, *, #11818, .F. ) ;
#16100=DIRECTION ( 'NONE',  ( 0.000000000000000000, 0.000000000000000000, -1.000000000000000000 ) ) ;
#16132=CARTESIAN_POINT ( 'NONE',  ( 11.00000000000000355, 26.00000000000000355, -87.20294101747086302 ) ) ;
#16149=DIRECTION ( 'NONE',  ( 0.000000000000000000, -0.000000000000000000, 1.000000000000000000 ) ) ;
#16152=VERTEX_POINT ( 'NONE', #27683 ) ;
#16167=CARTESIAN_POINT ( 'NONE',  ( -52.00000000000001421, 2.499999999999999556, -60.00000000000000000 ) ) ;
#16194=CARTESIAN_POINT ( 'NONE',  ( 33.00000000000001421, -4.500000000000000000, 40.00000000000002842 ) ) ;
#16223=FACE_OUTER_BOUND ( 'NONE', #24204, .T. ) ;
#16253=ADVANCED_FACE ( 'NONE', ( #2367 ), #18117, .F. ) ;
#16273=DIRECTION ( 'NONE',  ( -0.000000000000000000, 1.000000000000000000, -0.000000000000000000 ) ) ;
#16294=ORIENTED_EDGE ( 'NONE', *, *, #39643, .F. ) ;
#16295=ORIENTED_EDGE ( 'NONE', *, *, #28713, .F. ) ;
#16298=CARTESIAN_POINT ( 'NONE',  ( 33.00000000000001421, -4.500000000000000000, 40.00000000000002842 ) ) ;
#16307=EDGE_CURVE ( 'NONE', #13199, #6143, #8845, .T. ) ;
#16316=VECTOR ( 'NONE', #27424, 1000.000000000000000 ) ;
#16347=EDGE_CURVE ( 'NONE', #38619, #5872, #28098, .T. ) ;
#16349=LINE ( 'NONE', #13778, #23966 ) ;
#16352=VERTEX_POINT ( 'NONE', #2148 ) ;
#16395=EDGE_CURVE ( 'NONE', #20097, #39331, #24925, .T. ) ;
#16416=CARTESIAN_POINT ( 'NONE',  ( 42.01694176638639533, -7.546903773697116513, 42.59507890604732694 ) ) ;
#16424=DIRECTION ( 'NONE',  ( -0.000000000000000000, 1.000000000000000000, -0.000000000000000000 ) ) ;
#16441=VERTEX_POINT ( 'NONE', #31499 ) ;
#16452=CIRCLE ( 'NONE', #11023, 10.00000000000000178 ) ;
#16458=DIRECTION ( 'NONE',  ( 1.000000000000000000, -0.000000000000000000, 0.000000000000000000 ) ) ;
#16478=CARTESIAN_POINT ( 'NONE',  ( 44.99999999999998579, -10.00000000000000000, 60.00000000000002132 ) ) ;
#16482=VERTEX_POINT ( 'NONE', #15357 ) ;
#16539=CARTESIAN_POINT ( 'NONE',  ( -49.99999999999998579, 2.499999999999999556, 55.00000000000002132 ) ) ;
#16544=CARTESIAN_POINT ( 'NONE',  ( -48.00000000000001421, -4.500000000000000000, 40.00000000000002842 ) ) ;
#16545=LINE ( 'NONE', #17171, #38981 ) ;
#16557=LINE ( 'NONE', #19526, #19871 ) ;
#16561=EDGE_LOOP ( 'NONE', ( #18644, #15763, #808, #13128 ) ) ;
#16576=FACE_OUTER_BOUND ( 'NONE', #26543, .T. ) ;
#16590=EDGE_CURVE ( 'NONE', #4135, #5569, #39130, .T. ) ;
#16612=ORIENTED_EDGE ( 'NONE', *, *, #646, .T. ) ;
#16619=CARTESIAN_POINT ( 'NONE',  ( 41.84926701758181622, -7.465541532174101214, 42.68631999426528267 ) ) ;
#16731=DIRECTION ( 'NONE',  ( -1.000000000000000000, 0.000000000000000000, 0.000000000000000000 ) ) ;
#16743=ORIENTED_EDGE ( 'NONE', *, *, #21049, .T. ) ;
#16764=ORIENTED_EDGE ( 'NONE', *, *, #6925, .F. ) ;
#16775=EDGE_CURVE ( 'NONE', #3829, #16352, #6653, .T. ) ;
#16817=EDGE_LOOP ( 'NONE', ( #11314, #17283, #15982, #29353, #10222 ) ) ;
#16819=EDGE_LOOP ( 'NONE', ( #5554, #30196, #6488, #32575 ) ) ;
#16826=CARTESIAN_POINT ( 'NONE',  ( 42.74543598854582171, -7.968564735797307286, 38.00154773414779186 ) ) ;
#16835=DIRECTION ( 'NONE',  ( 0.000000000000000000, 0.000000000000000000, -1.000000000000000000 ) ) ;
#16859=EDGE_CURVE ( 'NONE', #626, #34897, #22973, .T. ) ;
#16861=EDGE_CURVE ( 'NONE', #27773, #18220, #14414, .T. ) ;
#16867=ADVANCED_FACE ( 'NONE', ( #7831 ), #33774, .T. ) ;
#16904=DIRECTION ( 'NONE',  ( 0.000000000000000000, 0.000000000000000000, -1.000000000000000000 ) ) ;
#16918=ADVANCED_FACE ( 'NONE', ( #18434 ), #24832, .F. ) ;
#16941=CARTESIAN_POINT ( 'NONE',  ( 44.99999999999999289, 10.00000000000000000, 55.00000000000002132 ) ) ;
#16950=ORIENTED_EDGE ( 'NONE', *, *, #39829, .F. ) ;
#16977=AXIS2_PLACEMENT_3D ( 'NONE', #29497, #39274, #29923 ) ;
#17010=AXIS2_PLACEMENT_3D ( 'NONE', #9683, #16273, #13479 ) ;
#17030=EDGE_CURVE ( 'NONE', #18435, #30146, #8858, .T. ) ;
#17038=CARTESIAN_POINT ( 'NONE',  ( 42.02078887490317527, -7.548854780837803702, 37.40723666453779828 ) ) ;
#17046=CARTESIAN_POINT ( 'NONE',  ( 40.50000000000000711, -15.00000000000000000, 40.00000000000002842 ) ) ;
#17065=EDGE_CURVE ( 'NONE', #40859, #9283, #12254, .T. ) ;
#17074=DIRECTION ( 'NONE',  ( 1.000000000000000000, -0.000000000000000000, 0.000000000000000000 ) ) ;
#17081=ORIENTED_EDGE ( 'NONE', *, *, #8264, .T. ) ;
#17092=EDGE_CURVE ( 'NONE', #37769, #22137, #22043, .T. ) ;
#17113=EDGE_CURVE ( 'NONE', #895, #18435, #5881, .T. ) ;
#17130=LINE ( 'NONE', #20947, #38081 ) ;
#17146=LINE ( 'NONE', #4383, #22079 ) ;
#17171=CARTESIAN_POINT ( 'NONE',  ( 47.99999999999998579, -10.00000000000000000, 0.000000000000000000 ) ) ;
#17190=VECTOR ( 'NONE', #8350, 1000.000000000000000 ) ;
#17209=CARTESIAN_POINT ( 'NONE',  ( 49.99999999999998579, 2.499999999999999556, 55.00000000000002132 ) ) ;
#17213=FACE_OUTER_BOUND ( 'NONE', #10896, .T. ) ;
#17215=DIRECTION ( 'NONE',  ( 1.000000000000000000, 0.000000000000000000, -0.000000000000000000 ) ) ;
#17236=ORIENTED_EDGE ( 'NONE', *, *, #19160, .F. ) ;
#17274=ORIENTED_EDGE ( 'NONE', *, *, #28530, .F. ) ;
#17279=VERTEX_POINT ( 'NONE', #28833 ) ;
#17283=ORIENTED_EDGE ( 'NONE', *, *, #39229, .F. ) ;
#17295=CARTESIAN_POINT ( 'NONE',  ( 52.00000000000002842, -2.499999999999999556, 60.00000000000002132 ) ) ;
#17309=AXIS2_PLACEMENT_3D ( 'NONE', #34972, #28371, #8602 ) ;
#17326=CARTESIAN_POINT ( 'NONE',  ( 40.29235768445109755, -7.145751311064569400, 43.00000000000005684 ) ) ;
#17421=LINE ( 'NONE', #1458, #41741 ) ;
#17468=CARTESIAN_POINT ( 'NONE',  ( -48.00000000000001421, 7.999999999999996447, 50.00000000000002842 ) ) ;
#17505=CARTESIAN_POINT ( 'NONE',  ( 40.50000000000000711, -15.00000000000000000, 44.00000000000004263 ) ) ;
#17538=VECTOR ( 'NONE', #26931, 1000.000000000000000 ) ;
#17568=EDGE_CURVE ( 'NONE', #29446, #37476, #17130, .T. ) ;
#17576=CARTESIAN_POINT ( 'NONE',  ( -11.00000000000000355, 10.00000000000000000, -59.99999999999999289 ) ) ;
#17593=AXIS2_PLACEMENT_3D ( 'NONE', #33440, #29822, #687 ) ;
#17611=ORIENTED_EDGE ( 'NONE', *, *, #13150, .F. ) ;
#17624=CARTESIAN_POINT ( 'NONE',  ( 40.50000000000000711, -15.00000000000000000, 40.00000000000002842 ) ) ;
#17638=CARTESIAN_POINT ( 'NONE',  ( 0.000000000000000000, -10.00000000000000000, -57.99999999999998579 ) ) ;
#17705=CIRCLE ( 'NONE', #3453, 10.00000000000000178 ) ;
#17709=DIRECTION ( 'NONE',  ( 1.000000000000000000, 0.000000000000000000, 0.000000000000000000 ) ) ;
#17740=CARTESIAN_POINT ( 'NONE',  ( 38.67128100893594222, -7.713523715135235825, 37.61436040636648670 ) ) ;
#17761=CARTESIAN_POINT ( 'NONE',  ( -52.00000000000002842, 10.00000000000000000, 60.00000000000002132 ) ) ;
#17764=LINE ( 'NONE', #1804, #10828 ) ;
#17788=ORIENTED_EDGE ( 'NONE', *, *, #13148, .F. ) ;
#17804=VERTEX_POINT ( 'NONE', #2215 ) ;
#17810=EDGE_CURVE ( 'NONE', #25504, #38216, #37945, .T. ) ;
#17812=DIRECTION ( 'NONE',  ( 0.000000000000000000, -0.000000000000000000, 1.000000000000000000 ) ) ;
#17821=VECTOR ( 'NONE', #34772, 1000.000000000000000 ) ;
#17847=PLANE ( 'NONE',  #30723 ) ;
#17852=DIRECTION ( 'NONE',  ( 0.000000000000000000, 0.000000000000000000, -1.000000000000000000 ) ) ;
#17854=AXIS2_PLACEMENT_3D ( 'NONE', #34123, #37122, #40510 ) ;
#17856=ORIENTED_EDGE ( 'NONE', *, *, #24611, .F. ) ;
#17862=ORIENTED_EDGE ( 'NONE', *, *, #6925, .T. ) ;
#17873=VECTOR ( 'NONE', #22796, 1000.000000000000000 ) ;
#17987=DIRECTION ( 'NONE',  ( 0.000000000000000000, -1.000000000000000000, 0.000000000000000000 ) ) ;
#18029=PRODUCT_DEFINITION_FORMATION_WITH_SPECIFIED_SOURCE ( 'ANY', '', #40444, .NOT_KNOWN. ) ;
#18032=FACE_OUTER_BOUND ( 'NONE', #34604, .T. ) ;
#18060=CARTESIAN_POINT ( 'NONE',  ( -33.00000000000001421, -4.500000000000000000, 40.00000000000002842 ) ) ;
#18105=EDGE_LOOP ( 'NONE', ( #31701, #5514, #27228, #21982, #31651, #41515, #34816, #7017 ) ) ;
#18117=CYLINDRICAL_SURFACE ( 'NONE', #19716, 3.000000000000002665 ) ;
#18122=DIRECTION ( 'NONE',  ( 1.000000000000000000, -0.000000000000000000, -0.000000000000000000 ) ) ;
#18152=ORIENTED_EDGE ( 'NONE', *, *, #11, .T. ) ;
#18156=FACE_OUTER_BOUND ( 'NONE', #16819, .T. ) ;
#18160=DIRECTION ( 'NONE',  ( -0.000000000000000000, -1.000000000000000000, -0.000000000000000000 ) ) ;
#18168=EDGE_CURVE ( 'NONE', #13040, #5872, #33079, .T. ) ;
#18182=DIRECTION ( 'NONE',  ( 0.000000000000000000, -1.000000000000000000, 0.000000000000000000 ) ) ;
#18188=FACE_OUTER_BOUND ( 'NONE', #32973, .T. ) ;
#18193=ADVANCED_FACE ( 'NONE', ( #33290 ), #10335, .T. ) ;
#18220=VERTEX_POINT ( 'NONE', #26925 ) ;
#18222=CARTESIAN_POINT ( 'NONE',  ( 40.50000000000000711, 10.00099999999999945, 43.00000000000004263 ) ) ;
#18237=FACE_OUTER_BOUND ( 'NONE', #29037, .T. ) ;
#18250=CARTESIAN_POINT ( 'NONE',  ( 48.00000000000001421, -10.00000000000000000, 48.35164654424506381 ) ) ;
#18270=DIRECTION ( 'NONE',  ( -0.000000000000000000, -1.000000000000000000, -0.000000000000000000 ) ) ;
#18271=AXIS2_PLACEMENT_3D ( 'NONE', #42028, #35634, #32436 ) ;
#18324=EDGE_CURVE ( 'NONE', #32782, #9431, #6173, .T. ) ;
#18331=ORIENTED_EDGE ( 'NONE', *, *, #16029, .T. ) ;
#18347=CARTESIAN_POINT ( 'NONE',  ( 40.50000000000000711, -10.00000000000000000, 40.00000000000002842 ) ) ;
#18348=DIRECTION ( 'NONE',  ( 0.000000000000000000, -0.000000000000000000, -1.000000000000000000 ) ) ;
#18349=CARTESIAN_POINT ( 'NONE',  ( 52.00000000000002842, 2.499999999999999556, 60.00000000000002132 ) ) ;
#18358=ADVANCED_FACE ( 'NONE', ( #37536 ), #40935, .T. ) ;
#18429=ORIENTED_EDGE ( 'NONE', *, *, #8544, .F. ) ;
#18434=FACE_OUTER_BOUND ( 'NONE', #23009, .T. ) ;
#18435=VERTEX_POINT ( 'NONE', #37134 ) ;
#18449=DIRECTION ( 'NONE',  ( 0.000000000000000000, -0.000000000000000000, -1.000000000000000000 ) ) ;
#18470=DIRECTION ( 'NONE',  ( 1.000000000000000000, 0.000000000000000000, 0.000000000000000000 ) ) ;
#18475=CARTESIAN_POINT ( 'NONE',  ( 33.00000000000001421, 7.999999999999996447, 50.00000000000002842 ) ) ;
#18481=VECTOR ( 'NONE', #10470, 1000.000000000000000 ) ;
#18483=ADVANCED_FACE ( 'NONE', ( #28374 ), #22412, .T. ) ;
#18515=LINE ( 'NONE', #5541, #1632 ) ;
#18539=ORIENTED_EDGE ( 'NONE', *, *, #27527, .T. ) ;
#18544=EDGE_CURVE ( 'NONE', #37469, #13206, #25411, .T. ) ;
#18573=LINE ( 'NONE', #31126, #32560 ) ;
#18574=CLOSED_SHELL ( 'NONE', ( #16918, #27420, #19366, #22101, #39337, #26092, #26702, #15302, #13945, #34867, #8433, #2484, #9475, #40012, #6442, #4126, #13402, #19102, #18483, #2466, #32865, #12946, #932, #31653, #31809, #204, #4814, #14005, #33463, #26772, #38093, #32131, #38415, #14453, #16253, #41733, #32797, #29052, #36654, #18888, #13667, #9923, #6683, #18193, #13332, #18358, #27929, #34586, #41471, #8276, #14921, #37641, #10080, #30630, #32325, #26914, #7979, #14267, #6606, #33042, #31989, #16867, #1234, #34148, #30522, #15530 ) ) ;
#18613=CARTESIAN_POINT ( 'NONE',  ( 33.00000000000001421, -4.500000000000000000, 36.00000000000002842 ) ) ;
#18617=CARTESIAN_POINT ( 'NONE',  ( 44.99999999999998579, 8.000000000000000000, 58.00000000000001421 ) ) ;
#18629=LINE ( 'NONE', #40963, #1645 ) ;
#18644=ORIENTED_EDGE ( 'NONE', *, *, #8190, .F. ) ;
#18648=CARTESIAN_POINT ( 'NONE',  ( -33.00000000000001421, 8.000000000000000000, 30.00000000000002132 ) ) ;
#18649=AXIS2_PLACEMENT_3D ( 'NONE', #32474, #29483, #22905 ) ;
#18680=CARTESIAN_POINT ( 'NONE',  ( -33.00000000000001421, -4.500000000000000000, 40.00000000000002842 ) ) ;
#18685=LINE ( 'NONE', #21653, #6941 ) ;
#18689=ORIENTED_EDGE ( 'NONE', *, *, #31551, .T. ) ;
#18694=ORIENTED_EDGE ( 'NONE', *, *, #9495, .T. ) ;
#18697=VECTOR ( 'NONE', #21574, 1000.000000000000000 ) ;
#18734=ORIENTED_EDGE ( 'NONE', *, *, #10009, .T. ) ;
#18772=LINE ( 'NONE', #32367, #25317 ) ;
#18783=ORIENTED_EDGE ( 'NONE', *, *, #25410, .T. ) ;
#18786=FACE_OUTER_BOUND ( 'NONE', #35896, .T. ) ;
#18796=ORIENTED_EDGE ( 'NONE', *, *, #18324, .F. ) ;
#18848=VERTEX_POINT ( 'NONE', #30320 ) ;
#18852=CARTESIAN_POINT ( 'NONE',  ( -33.00000000000001421, -4.500000000000000000, 30.00000000000002842 ) ) ;
#18885=LINE ( 'NONE', #29281, #11527 ) ;
#18888=ADVANCED_FACE ( 'NONE', ( #28173 ), #41576, .F. ) ;
#18902=DIRECTION ( 'NONE',  ( -0.000000000000000000, 1.000000000000000000, -0.000000000000000000 ) ) ;
#18962=ORIENTED_EDGE ( 'NONE', *, *, #5949, .F. ) ;
#18981=DIRECTION ( 'NONE',  ( 0.000000000000000000, -1.000000000000000000, 0.000000000000000000 ) ) ;
#19015=VECTOR ( 'NONE', #20677, 1000.000000000000000 ) ;
#19024=DIRECTION ( 'NONE',  ( 0.000000000000000000, 0.000000000000000000, -1.000000000000000000 ) ) ;
#19041=EDGE_LOOP ( 'NONE', ( #23568, #39560, #25642, #27899 ) ) ;
#19061=CARTESIAN_POINT ( 'NONE',  ( -73.31370849898480913, -4.499999999999999112, 44.00000000000003553 ) ) ;
#19065=VECTOR ( 'NONE', #1727, 1000.000000000000000 ) ;
#19080=CARTESIAN_POINT ( 'NONE',  ( -45.00000000000002132, -10.00000000000000000, 58.00000000000002132 ) ) ;
#19102=ADVANCED_FACE ( 'NONE', ( #32409 ), #36011, .T. ) ;
#19119=DIRECTION ( 'NONE',  ( 0.000000000000000000, 0.000000000000000000, -1.000000000000000000 ) ) ;
#19160=EDGE_CURVE ( 'NONE', #895, #38619, #22416, .T. ) ;
#19163=FACE_OUTER_BOUND ( 'NONE', #836, .T. ) ;
#19167=CARTESIAN_POINT ( 'NONE',  ( -33.00000000000001421, -4.500000000000000000, 36.00000000000002842 ) ) ;
#19183=CARTESIAN_POINT ( 'NONE',  ( 62.00000000000001421, 2.499999999999999556, -49.99999999999998579 ) ) ;
#19262=ORIENTED_EDGE ( 'NONE', *, *, #1262, .T. ) ;
#19347=CARTESIAN_POINT ( 'NONE',  ( 48.00000000000001421, -4.500000000000000000, 30.00000000000002842 ) ) ;
#19366=ADVANCED_FACE ( 'NONE', ( #10077, #23043 ), #496, .F. ) ;
#19375=EDGE_LOOP ( 'NONE', ( #16, #261, #30569, #32073 ) ) ;
#19396=VERTEX_POINT ( 'NONE', #29843 ) ;
#19416=DIRECTION ( 'NONE',  ( 1.000000000000000000, 0.000000000000000000, -0.000000000000000000 ) ) ;
#19454=CYLINDRICAL_SURFACE ( 'NONE', #17010, 4.000000000000010658 ) ;
#19468=FACE_OUTER_BOUND ( 'NONE', #35489, .T. ) ;
#19475=EDGE_LOOP ( 'NONE', ( #10539, #11456, #4876, #26177 ) ) ;
#19515=DIRECTION ( 'NONE',  ( 0.000000000000000000, 1.000000000000000000, 0.000000000000000000 ) ) ;
#19526=CARTESIAN_POINT ( 'NONE',  ( 33.00000000000001421, -10.00000000000000000, 31.64835345575499304 ) ) ;
#19529=ORIENTED_EDGE ( 'NONE', *, *, #25736, .F. ) ;
#19552=CARTESIAN_POINT ( 'NONE',  ( 47.99999999999998579, 10.00000000000000000, 60.00000000000002132 ) ) ;
#19566=ORIENTED_EDGE ( 'NONE', *, *, #23153, .F. ) ;
#19574=ORIENTED_EDGE ( 'NONE', *, *, #26182, .T. ) ;
#19588=LINE ( 'NONE', #3636, #34141 ) ;
#19604=DIRECTION ( 'NONE',  ( 0.000000000000000000, -1.000000000000000000, 0.000000000000000000 ) ) ;
#19639=DIRECTION ( 'NONE',  ( 0.000000000000000000, 0.000000000000000000, -1.000000000000000000 ) ) ;
#19657=ORIENTED_EDGE ( 'NONE', *, *, #25665, .F. ) ;
#19672=ORIENTED_EDGE ( 'NONE', *, *, #35925, .T. ) ;
#19688=DIRECTION ( 'NONE',  ( 0.000000000000000000, 0.000000000000000000, 1.000000000000000000 ) ) ;
#19707=LINE ( 'NONE', #29267, #25846 ) ;
#19714=FACE_OUTER_BOUND ( 'NONE', #21236, .T. ) ;
#19716=AXIS2_PLACEMENT_3D ( 'NONE', #40864, #34277, #41290 ) ;
#19735=CIRCLE ( 'NONE', #13621, 10.00000000000000178 ) ;
#19744=EDGE_CURVE ( 'NONE', #31075, #5294, #20228, .T. ) ;
#19757=VECTOR ( 'NONE', #246, 1000.000000000000000 ) ;
#19776=CARTESIAN_POINT ( 'NONE',  ( -33.00000000000001421, 8.000000000000000000, 30.00000000000002132 ) ) ;
#19778=ORIENTED_EDGE ( 'NONE', *, *, #3118, .F. ) ;
#19799=DIRECTION ( 'NONE',  ( 0.000000000000000000, 0.000000000000000000, -1.000000000000000000 ) ) ;
#19815=ORIENTED_EDGE ( 'NONE', *, *, #37424, .T. ) ;
#19841=LINE ( 'NONE', #13459, #2716 ) ;
#19868=CIRCLE ( 'NONE', #26681, 10.00000000000000178 ) ;
#19871=VECTOR ( 'NONE', #26758, 1000.000000000000000 ) ;
#19874=VECTOR ( 'NONE', #7339, 1000.000000000000000 ) ;
#19877=FACE_BOUND ( 'NONE', #22450, .T. ) ;
#19879=SHAPE_DEFINITION_REPRESENTATION ( #10893, #29355 ) ;
#19882=EDGE_CURVE ( 'NONE', #11057, #40914, #21274, .T. ) ;
#19885=EDGE_CURVE ( 'NONE', #25917, #13040, #20508, .T. ) ;
#19899=DIRECTION ( 'NONE',  ( 0.000000000000000000, 0.000000000000000000, -1.000000000000000000 ) ) ;
#19908=AXIS2_PLACEMENT_3D ( 'NONE', #31661, #18270, #21463 ) ;
#19943=ORIENTED_EDGE ( 'NONE', *, *, #23011, .F. ) ;
#19950=ORIENTED_EDGE ( 'NONE', *, *, #15039, .T. ) ;
#19955=CIRCLE ( 'NONE', #1612, 4.999999999999984013 ) ;
#19969=FACE_OUTER_BOUND ( 'NONE', #30084, .T. ) ;
#19998=AXIS2_PLACEMENT_3D ( 'NONE', #604, #10399, #33142 ) ;
#20004=EDGE_LOOP ( 'NONE', ( #39991, #28606, #7859, #2110 ) ) ;
#20015=CARTESIAN_POINT ( 'NONE',  ( 40.91198259643069690, -7.170723060291307682, 42.97840118858466951 ) ) ;
#20036=ORIENTED_EDGE ( 'NONE', *, *, #13942, .T. ) ;
#20040=CARTESIAN_POINT ( 'NONE',  ( 33.00000000000001421, -4.500000000000000000, 30.00000000000002842 ) ) ;
#20097=VERTEX_POINT ( 'NONE', #10813 ) ;
#20134=LINE ( 'NONE', #10352, #12198 ) ;
#20135=LINE ( 'NONE', #36077, #31541 ) ;
#20142=ORIENTED_EDGE ( 'NONE', *, *, #17810, .F. ) ;
#20163=ORIENTED_EDGE ( 'NONE', *, *, #25760, .T. ) ;
#20167=EDGE_CURVE ( 'NONE', #5504, #1841, #7846, .T. ) ;
#20185=EDGE_CURVE ( 'NONE', #30146, #3829, #20389, .T. ) ;
#20201=ORIENTED_EDGE ( 'NONE', *, *, #4337, .T. ) ;
#20228=LINE ( 'NONE', #10868, #13700 ) ;
#20234=EDGE_CURVE ( 'NONE', #40914, #27545, #27286, .T. ) ;
#20260=ORIENTED_EDGE ( 'NONE', *, *, #9495, .F. ) ;
#20261=DIRECTION ( 'NONE',  ( 0.000000000000000000, 0.000000000000000000, -1.000000000000000000 ) ) ;
#20278=VECTOR ( 'NONE', #33431, 1000.000000000000000 ) ;
#20287=LINE ( 'NONE', #23915, #23311 ) ;
#20309=CIRCLE ( 'NONE', #7411, 3.000000000000002665 ) ;
#20354=CARTESIAN_POINT ( 'NONE',  ( -48.00000000000001421, -4.500000000000000000, 30.00000000000002842 ) ) ;
#20378=CIRCLE ( 'NONE', #40078, 4.999999999999997335 ) ;
#20389=LINE ( 'NONE', #11030, #24577 ) ;
#20397=DIRECTION ( 'NONE',  ( 0.000000000000000000, -1.000000000000000000, 0.000000000000000000 ) ) ;
#20420=EDGE_CURVE ( 'NONE', #16039, #18220, #31628, .T. ) ;
#20472=PLANE ( 'NONE',  #17593 ) ;
#20479=DIRECTION ( 'NONE',  ( 0.000000000000000000, 0.000000000000000000, 1.000000000000000000 ) ) ;
#20504=CARTESIAN_POINT ( 'NONE',  ( 10.00000000000000178, 10.00000000000000000, -59.99999999999999289 ) ) ;
#20508=CIRCLE ( 'NONE', #30675, 3.000000000000002665 ) ;
#20510=CARTESIAN_POINT ( 'NONE',  ( 40.29159080925865766, -7.145751311064597822, 37.00000000000002132 ) ) ;
#20556=CIRCLE ( 'NONE', #38921, 4.000000000000003553 ) ;
#20570=CARTESIAN_POINT ( 'NONE',  ( -33.00000000000001421, -10.00000000000000000, 31.64835345575499304 ) ) ;
#20610=DIRECTION ( 'NONE',  ( 0.000000000000000000, -1.000000000000000000, 0.000000000000000000 ) ) ;
#20613=VERTEX_POINT ( 'NONE', #19080 ) ;
#20624=CIRCLE ( 'NONE', #5577, 10.00000000000000178 ) ;
#20665=DIRECTION ( 'NONE',  ( 0.000000000000000000, -1.000000000000000000, 5.551115123125782702E-16 ) ) ;
#20677=DIRECTION ( 'NONE',  ( 0.000000000000000000, 0.000000000000000000, -1.000000000000000000 ) ) ;
#20685=CIRCLE ( 'NONE', #18649, 10.00000000000000178 ) ;
#20709=VECTOR ( 'NONE', #25562, 1000.000000000000000 ) ;
#20715=VECTOR ( 'NONE', #14987, 1000.000000000000000 ) ;
#20727=DIRECTION ( 'NONE',  ( 0.000000000000000000, 0.000000000000000000, -1.000000000000000000 ) ) ;
#20770=EDGE_CURVE ( 'NONE', #27620, #6143, #3956, .T. ) ;
#20787=DIRECTION ( 'NONE',  ( -1.000000000000000000, 0.000000000000000000, 1.067522139062650178E-16 ) ) ;
#20806=VECTOR ( 'NONE', #38304, 1000.000000000000000 ) ;
#20824=CARTESIAN_POINT ( 'NONE',  ( -45.00000000000002132, -10.00000000000000000, -55.00000000000000000 ) ) ;
#20832=CARTESIAN_POINT ( 'NONE',  ( -45.00000000000002132, 10.00000000000000000, 60.00000000000002132 ) ) ;
#20902=EDGE_CURVE ( 'NONE', #40357, #7819, #13959, .T. ) ;
#20931=CARTESIAN_POINT ( 'NONE',  ( 37.60631596752138961, -8.420793647684782002, 39.18284160825089657 ) ) ;
#20947=CARTESIAN_POINT ( 'NONE',  ( 10.00000000000000178, 25.00000000000000000, 60.00000000000002132 ) ) ;
#20952=CARTESIAN_POINT ( 'NONE',  ( -9.999999999999998224, 25.00000000000000000, -59.99999999999999289 ) ) ;
#20954=AXIS2_PLACEMENT_3D ( 'NONE', #41127, #25387, #2828 ) ;
#20955=EDGE_CURVE ( 'NONE', #21502, #33064, #556, .T. ) ;
#20968=CARTESIAN_POINT ( 'NONE',  ( -45.00000000000002132, -2.500000000000000444, -59.99999999999999289 ) ) ;
#21001=DIRECTION ( 'NONE',  ( 0.000000000000000000, 1.000000000000000000, 0.000000000000000000 ) ) ;
#21018=CARTESIAN_POINT ( 'NONE',  ( 52.00000000000002132, -2.499999999999999556, -60.00000000000000000 ) ) ;
#21022=DIRECTION ( 'NONE',  ( 1.000000000000000000, 0.000000000000000000, 0.000000000000000000 ) ) ;
#21038=FACE_OUTER_BOUND ( 'NONE', #12351, .T. ) ;
#21049=EDGE_CURVE ( 'NONE', #19396, #1429, #36091, .T. ) ;
#21069=VECTOR ( 'NONE', #10767, 1000.000000000000000 ) ;
#21086=ORIENTED_EDGE ( 'NONE', *, *, #5913, .F. ) ;
#21156=EDGE_CURVE ( 'NONE', #36692, #26597, #30344, .T. ) ;
#21158=EDGE_CURVE ( 'NONE', #34897, #15972, #14185, .T. ) ;
#21193=EDGE_CURVE ( 'NONE', #11983, #40859, #28664, .T. ) ;
#21218=ORIENTED_EDGE ( 'NONE', *, *, #27480, .F. ) ;
#21219=AXIS2_PLACEMENT_3D ( 'NONE', #2449, #28599, #40950 ) ;
#21224=CARTESIAN_POINT ( 'NONE',  ( -10.00000000000000178, 10.00000000000000000, -59.99999999999999289 ) ) ;
#21236=EDGE_LOOP ( 'NONE', ( #35572, #12243, #33971, #27419 ) ) ;
#21240=DIRECTION ( 'NONE',  ( -0.000000000000000000, -1.000000000000000000, 0.000000000000000000 ) ) ;
#21247=CARTESIAN_POINT ( 'NONE',  ( -45.00000000000002132, -2.499999999999999556, -55.00000000000000000 ) ) ;
#21254=ORIENTED_EDGE ( 'NONE', *, *, #8607, .F. ) ;
#21274=LINE ( 'NONE', #37441, #33400 ) ;
#21354=ORIENTED_EDGE ( 'NONE', *, *, #10535, .F. ) ;
#21363=AXIS2_PLACEMENT_3D ( 'NONE', #17624, #23801, #40578 ) ;
#21376=DIRECTION ( 'NONE',  ( 0.000000000000000000, -1.000000000000000000, 0.000000000000000000 ) ) ;
#21402=VECTOR ( 'NONE', #8450, 1000.000000000000000 ) ;
#21451=DIRECTION ( 'NONE',  ( 0.000000000000000000, -1.000000000000000000, 0.000000000000000000 ) ) ;
#21463=DIRECTION ( 'NONE',  ( 0.000000000000000000, 0.000000000000000000, 1.000000000000000000 ) ) ;
#21485=CIRCLE ( 'NONE', #22857, 4.000000000000003553 ) ;
#21494=DIRECTION ( 'NONE',  ( 1.000000000000000000, -0.000000000000000000, -0.000000000000000000 ) ) ;
#21502=VERTEX_POINT ( 'NONE', #31795 ) ;
#21513=DIRECTION ( 'NONE',  ( 0.000000000000000000, -1.000000000000000000, 0.000000000000000000 ) ) ;
#21552=PLANE ( 'NONE',  #21733 ) ;
#21567=CARTESIAN_POINT ( 'NONE',  ( -45.00000000000002132, 10.00000000000000000, -59.99999999999999289 ) ) ;
#21574=DIRECTION ( 'NONE',  ( -1.000000000000000000, -0.000000000000000000, -0.000000000000000000 ) ) ;
#21589=CYLINDRICAL_SURFACE ( 'NONE', #38860, 4.999999999999997335 ) ;
#21617=DIRECTION ( 'NONE',  ( 1.000000000000000000, -0.000000000000000000, -1.067522139062650178E-16 ) ) ;
#21630=DIRECTION ( 'NONE',  ( 0.000000000000000000, 0.000000000000000000, -1.000000000000000000 ) ) ;
#21649=CARTESIAN_POINT ( 'NONE',  ( 33.00000000000001421, -4.500000000000000000, 30.00000000000002842 ) ) ;
#21653=CARTESIAN_POINT ( 'NONE',  ( -50.00000000000001421, 10.00000000000000000, 55.00000000000002132 ) ) ;
#21661=VERTEX_POINT ( 'NONE', #26650 ) ;
#21668=ORIENTED_EDGE ( 'NONE', *, *, #16029, .F. ) ;
#21683=DIRECTION ( 'NONE',  ( -0.000000000000000000, 1.000000000000000000, -0.000000000000000000 ) ) ;
#21733=AXIS2_PLACEMENT_3D ( 'NONE', #11974, #8578, #24968 ) ;
#21746=CARTESIAN_POINT ( 'NONE',  ( -45.00000000000002132, 8.000000000000000000, 58.00000000000001421 ) ) ;
#21767=AXIS2_PLACEMENT_3D ( 'NONE', #5009, #21805, #5222 ) ;
#21793=CIRCLE ( 'NONE', #31964, 10.00000000000000178 ) ;
#21805=DIRECTION ( 'NONE',  ( -0.000000000000000000, 1.000000000000000000, -0.000000000000000000 ) ) ;
#21828=ORIENTED_EDGE ( 'NONE', *, *, #37424, .F. ) ;
#21832=DIRECTION ( 'NONE',  ( -0.000000000000000000, -1.000000000000000000, -0.000000000000000000 ) ) ;
#21860=DIRECTION ( 'NONE',  ( 1.000000000000000000, 0.000000000000000000, 0.000000000000000000 ) ) ;
#21869=AXIS2_PLACEMENT_3D ( 'NONE', #8011, #2251, #41181 ) ;
#21901=LINE ( 'NONE', #19347, #7033 ) ;
#21937=VERTEX_POINT ( 'NONE', #34700 ) ;
#21965=VERTEX_POINT ( 'NONE', #10175 ) ;
#21982=ORIENTED_EDGE ( 'NONE', *, *, #24611, .T. ) ;
#21990=DIRECTION ( 'NONE',  ( 1.000000000000000000, 0.000000000000000000, 0.000000000000000000 ) ) ;
#22043=LINE ( 'NONE', #24618, #36003 ) ;
#22079=VECTOR ( 'NONE', #39896, 1000.000000000000000 ) ;
#22085=FACE_BOUND ( 'NONE', #28830, .T. ) ;
#22094=VECTOR ( 'NONE', #4782, 1000.000000000000000 ) ;
#22098=AXIS2_PLACEMENT_3D ( 'NONE', #41740, #25370, #32158 ) ;
#22101=ADVANCED_FACE ( 'NONE', ( #15564 ), #41514, .F. ) ;
#22119=DIRECTION ( 'NONE',  ( 0.000000000000000000, 1.000000000000000000, -5.551115123125782702E-16 ) ) ;
#22137=VERTEX_POINT ( 'NONE', #19167 ) ;
#22155=EDGE_CURVE ( 'NONE', #40605, #32782, #36754, .T. ) ;
#22166=LINE ( 'NONE', #39354, #11056 ) ;
#22173=LINE ( 'NONE', #6005, #11178 ) ;
#22237=ORIENTED_EDGE ( 'NONE', *, *, #32978, .F. ) ;
#22302=CARTESIAN_POINT ( 'NONE',  ( -73.31370849898480913, -4.500000000000000000, 40.00000000000002842 ) ) ;
#22317=FACE_OUTER_BOUND ( 'NONE', #33851, .T. ) ;
#22332=DIRECTION ( 'NONE',  ( 0.000000000000000000, -1.000000000000000000, 0.000000000000000000 ) ) ;
#22398=VECTOR ( 'NONE', #6550, 1000.000000000000000 ) ;
#22407=CARTESIAN_POINT ( 'NONE',  ( -62.00000000000001421, 2.499999999999999556, -60.00000000000000000 ) ) ;
#22412=CYLINDRICAL_SURFACE ( 'NONE', #5505, 4.999999999999997335 ) ;
#22416=LINE ( 'NONE', #35393, #8238 ) ;
#22432=VECTOR ( 'NONE', #32829, 1000.000000000000000 ) ;
#22450=EDGE_LOOP ( 'NONE', ( #3988, #36256, #31083, #26178 ) ) ;
#22453=DIRECTION ( 'NONE',  ( 1.000000000000000000, -0.000000000000000000, -0.000000000000000000 ) ) ;
#22539=ORIENTED_EDGE ( 'NONE', *, *, #21158, .T. ) ;
#22578=CIRCLE ( 'NONE', #9696, 10.00000000000000178 ) ;
#22597=CARTESIAN_POINT ( 'NONE',  ( -45.00000000000002132, -10.00000000000000000, -55.00000000000000000 ) ) ;
#22610=CIRCLE ( 'NONE', #875, 10.00000000000000178 ) ;
#22629=EDGE_CURVE ( 'NONE', #15408, #23612, #8788, .T. ) ;
#22645=DIRECTION ( 'NONE',  ( 0.000000000000000000, 0.000000000000000000, -1.000000000000000000 ) ) ;
#22731=VECTOR ( 'NONE', #11729, 1000.000000000000000 ) ;
#22772=EDGE_CURVE ( 'NONE', #5870, #33611, #17764, .T. ) ;
#22796=DIRECTION ( 'NONE',  ( -0.000000000000000000, -1.000000000000000000, -0.000000000000000000 ) ) ;
#22857=AXIS2_PLACEMENT_3D ( 'NONE', #12687, #32248, #10120 ) ;
#22866=PRODUCT_DEFINITION ( 'UNKNOWN', '', #18029, #341 ) ;
#22884=DIRECTION ( 'NONE',  ( -0.000000000000000000, -1.000000000000000000, -0.000000000000000000 ) ) ;
#22893=UNCERTAINTY_MEASURE_WITH_UNIT (LENGTH_MEASURE( 1.000000000000000082E-05 ), #10878, 'distance_accuracy_value', 'NONE');
#22905=DIRECTION ( 'NONE',  ( 0.000000000000000000, 0.000000000000000000, 1.000000000000000000 ) ) ;
#22973=LINE ( 'NONE', #4209, #26528 ) ;
#22975=CARTESIAN_POINT ( 'NONE',  ( 44.99999999999998579, -2.499999999999999556, -60.00000000000000000 ) ) ;
#22976=VECTOR ( 'NONE', #27320, 1000.000000000000000 ) ;
#22990=CARTESIAN_POINT ( 'NONE',  ( 40.50000000000000711, -7.145751311064596933, 37.00000000000001421 ) ) ;
#23009=EDGE_LOOP ( 'NONE', ( #29766, #20036, #30824, #26135 ) ) ;
#23010=CARTESIAN_POINT ( 'NONE',  ( -48.00000000000001421, -10.00000000000000000, 31.64835345575499304 ) ) ;
#23011=EDGE_CURVE ( 'NONE', #5504, #746, #2006, .T. ) ;
#23043=FACE_OUTER_BOUND ( 'NONE', #19041, .T. ) ;
#23060=ORIENTED_EDGE ( 'NONE', *, *, #21156, .F. ) ;
#23070=VECTOR ( 'NONE', #40801, 1000.000000000000000 ) ;
#23115=CARTESIAN_POINT ( 'NONE',  ( -11.00000000000000355, 26.00000000000000355, -59.99999999999999289 ) ) ;
#23143=VECTOR ( 'NONE', #21990, 1000.000000000000000 ) ;
#23148=DIRECTION ( 'NONE',  ( 0.000000000000000000, 1.000000000000000000, -0.000000000000000000 ) ) ;
#23153=EDGE_CURVE ( 'NONE', #903, #13780, #19841, .T. ) ;
#23156=EDGE_CURVE ( 'NONE', #626, #26542, #4075, .T. ) ;
#23185=CARTESIAN_POINT ( 'NONE',  ( -48.00000000000001421, 10.00000000000000000, 55.00000000000002132 ) ) ;
#23218=ORIENTED_EDGE ( 'NONE', *, *, #19744, .F. ) ;
#23242=EDGE_CURVE ( 'NONE', #30146, #17279, #36211, .T. ) ;
#23243=VECTOR ( 'NONE', #2655, 1000.000000000000000 ) ;
#23283=ORIENTED_EDGE ( 'NONE', *, *, #3799, .T. ) ;
#23311=VECTOR ( 'NONE', #10295, 1000.000000000000000 ) ;
#23329=CARTESIAN_POINT ( 'NONE',  ( -49.99999999999998579, -2.499999999999999556, -54.99999999999997158 ) ) ;
#23344=CARTESIAN_POINT ( 'NONE',  ( -48.00000000000001421, 10.00000000000000000, 60.00000000000002132 ) ) ;
#23357=ORIENTED_EDGE ( 'NONE', *, *, #34411, .F. ) ;
#23384=ORIENTED_EDGE ( 'NONE', *, *, #27480, .T. ) ;
#23404=ORIENTED_EDGE ( 'NONE', *, *, #16775, .F. ) ;
#23415=ORIENTED_EDGE ( 'NONE', *, *, #40439, .F. ) ;
#23431=LINE ( 'NONE', #13853, #41624 ) ;
#23497=CARTESIAN_POINT ( 'NONE',  ( 40.50000000000000711, -7.145751311064572064, 43.00000000000004263 ) ) ;
#23499=FACE_OUTER_BOUND ( 'NONE', #26174, .T. ) ;
#23514=CARTESIAN_POINT ( 'NONE',  ( -11.00000000000000355, 26.00000000000000355, -59.99999999999999289 ) ) ;
#23515=CARTESIAN_POINT ( 'NONE',  ( 44.99999999999998579, -10.00000000000000000, 58.00000000000001421 ) ) ;
#23537=AXIS2_PLACEMENT_3D ( 'NONE', #38470, #15084, #2317 ) ;
#23557=DIRECTION ( 'NONE',  ( 1.000000000000000000, 0.000000000000000000, 0.000000000000000000 ) ) ;
#23558=DIRECTION ( 'NONE',  ( 0.000000000000000000, 0.000000000000000000, -1.000000000000000000 ) ) ;
#23568=ORIENTED_EDGE ( 'NONE', *, *, #37280, .F. ) ;
#23605=DIRECTION ( 'NONE',  ( 0.000000000000000000, 0.000000000000000000, 1.000000000000000000 ) ) ;
#23612=VERTEX_POINT ( 'NONE', #4450 ) ;
#23616=ORIENTED_EDGE ( 'NONE', *, *, #4575, .T. ) ;
#23639=CARTESIAN_POINT ( 'NONE',  ( 43.33121732208139321, -8.374640936574810013, 41.01147694437517544 ) ) ;
#23686=( NAMED_UNIT ( * ) PLANE_ANGLE_UNIT ( ) SI_UNIT ( $, .RADIAN. ) );
#23693=AXIS2_PLACEMENT_3D ( 'NONE', #12726, #3357, #159 ) ;
#23707=ORIENTED_EDGE ( 'NONE', *, *, #29277, .T. ) ;
#23709=CARTESIAN_POINT ( 'NONE',  ( 37.91989015104953609, -8.194693614929777326, 38.45751407980970527 ) ) ;
#23728=EDGE_LOOP ( 'NONE', ( #1895, #6425 ) ) ;
#23744=DIRECTION ( 'NONE',  ( -1.000000000000000000, -0.000000000000000000, -0.000000000000000000 ) ) ;
#23764=CARTESIAN_POINT ( 'NONE',  ( -48.00000000000001421, -10.00000000000000000, 0.000000000000000000 ) ) ;
#23795=VECTOR ( 'NONE', #36971, 1000.000000000000000 ) ;
#23801=DIRECTION ( 'NONE',  ( 0.000000000000000000, -1.000000000000000000, 0.000000000000000000 ) ) ;
#23834=AXIS2_PLACEMENT_3D ( 'NONE', #27752, #18182, #14583 ) ;
#23837=CARTESIAN_POINT ( 'NONE',  ( -9.999999999999998224, 25.00000000000000000, 60.00000000000002132 ) ) ;
#23854=CARTESIAN_POINT ( 'NONE',  ( 43.33609834095070568, -8.378213985267427333, 39.00210443663780779 ) ) ;
#23915=CARTESIAN_POINT ( 'NONE',  ( -33.00000000000001421, -10.00000000000000000, 40.00000000000002842 ) ) ;
#23919=ORIENTED_EDGE ( 'NONE', *, *, #20234, .T. ) ;
#23922=DIRECTION ( 'NONE',  ( 0.000000000000000000, -0.000000000000000000, -1.000000000000000000 ) ) ;
#23923=CARTESIAN_POINT ( 'NONE',  ( 39.69116761968479068, -7.259815326113772116, 42.89605348060379697 ) ) ;
#23938=VERTEX_POINT ( 'NONE', #33430 ) ;
#23966=VECTOR ( 'NONE', #164, 1000.000000000000000 ) ;
#23971=AXIS2_PLACEMENT_3D ( 'NONE', #38622, #41196, #41830 ) ;
#23977=ORIENTED_EDGE ( 'NONE', *, *, #41025, .T. ) ;
#23985=LINE ( 'NONE', #37360, #40319 ) ;
#24000=CARTESIAN_POINT ( 'NONE',  ( -50.00000000000001421, 10.00000000000000000, -59.99999999999999289 ) ) ;
#24002=ORIENTED_EDGE ( 'NONE', *, *, #40975, .T. ) ;
#24051=ORIENTED_EDGE ( 'NONE', *, *, #1489, .F. ) ;
#24066=CARTESIAN_POINT ( 'NONE',  ( 62.00000000000002842, -4.500000000000000000, 40.00000000000001421 ) ) ;
#24112=DIRECTION ( 'NONE',  ( 0.000000000000000000, 0.000000000000000000, 1.000000000000000000 ) ) ;
#24140=EDGE_CURVE ( 'NONE', #12880, #40068, #33212, .T. ) ;
#24204=EDGE_LOOP ( 'NONE', ( #19950, #2839, #12980, #39389 ) ) ;
#24217=CARTESIAN_POINT ( 'NONE',  ( -48.00000000000001421, 10.00000000000000000, -54.99999999999997158 ) ) ;
#24220=DIRECTION ( 'NONE',  ( 0.000000000000000000, 0.000000000000000000, 1.000000000000000000 ) ) ;
#24241=DIRECTION ( 'NONE',  ( -0.000000000000000000, -1.000000000000000000, 0.000000000000000000 ) ) ;
#24291=B_SPLINE_CURVE_WITH_KNOTS ( 'NONE', 3,
 ( #7537, #20510, #37109, #27530, #33902, #37309, #33480, #17740, #39645, #949, #27104, #23709, #13703, #36891, #20931, #40072, #30289, #30497, #8162, #4345, #30714, #10516, #13915, #26894, #1367, #36460, #33260, #29282, #14342, #729, #23923, #27321, #17326, #23497 ),
 .UNSPECIFIED., .F., .F.,
 ( 4, 2, 2, 2, 2, 2, 2, 2, 2, 2, 2, 2, 2, 2, 2, 2, 4 ),
 ( 0.000000000000000000, 0.0006124279316953673644, 0.001224855863390734729, 0.001837283795086101876, 0.002449711726781469458, 0.003062139658476835304, 0.003674567590172201585, 0.004286995521867567431, 0.004899423453562934579, 0.005511851385258300859, 0.006124279316953666272, 0.006736707248649032552, 0.007349135180344398832, 0.007961563112039765980, 0.008573991043735131393, 0.009186418975430496806, 0.009798846907125863953 ),
 .UNSPECIFIED. ) ;
#24334=ORIENTED_EDGE ( 'NONE', *, *, #12235, .F. ) ;
#24355=EDGE_LOOP ( 'NONE', ( #15138, #12922, #29725, #25268, #10742, #1333, #19262, #37799 ) ) ;
#24384=ORIENTED_EDGE ( 'NONE', *, *, #21193, .T. ) ;
#24396=ORIENTED_EDGE ( 'NONE', *, *, #8745, .F. ) ;
#24402=ORIENTED_EDGE ( 'NONE', *, *, #4725, .F. ) ;
#24492=ORIENTED_EDGE ( 'NONE', *, *, #33336, .T. ) ;
#24528=LINE ( 'NONE', #37495, #17190 ) ;
#24540=CIRCLE ( 'NONE', #2789, 5.000000000000004441 ) ;
#24551=AXIS2_PLACEMENT_3D ( 'NONE', #15425, #24576, #5843 ) ;
#24557=VERTEX_POINT ( 'NONE', #4465 ) ;
#24558=ORIENTED_EDGE ( 'NONE', *, *, #13784, .F. ) ;
#24576=DIRECTION ( 'NONE',  ( 0.000000000000000000, 1.000000000000000000, 0.000000000000000000 ) ) ;
#24577=VECTOR ( 'NONE', #7627, 1000.000000000000000 ) ;
#24586=CARTESIAN_POINT ( 'NONE',  ( -48.00000000000001421, -4.500000000000000888, 50.00000000000002842 ) ) ;
#24611=EDGE_CURVE ( 'NONE', #34897, #31292, #33915, .T. ) ;
#24612=ORIENTED_EDGE ( 'NONE', *, *, #8264, .F. ) ;
#24618=CARTESIAN_POINT ( 'NONE',  ( -73.31370849898480913, -4.500000000000000000, 36.00000000000002842 ) ) ;
#24646=EDGE_CURVE ( 'NONE', #39773, #3291, #5399, .T. ) ;
#24662=VECTOR ( 'NONE', #5069, 1000.000000000000000 ) ;
#24687=PLANE ( 'NONE',  #40030 ) ;
#24744=AXIS2_PLACEMENT_3D ( 'NONE', #39961, #14443, #17215 ) ;
#24781=ORIENTED_EDGE ( 'NONE', *, *, #38589, .F. ) ;
#24811=CARTESIAN_POINT ( 'NONE',  ( 62.00000000000001421, 2.499999999999999556, -60.00000000000000000 ) ) ;
#24832=CYLINDRICAL_SURFACE ( 'NONE', #8175, 3.000000000000016431 ) ;
#24834=CARTESIAN_POINT ( 'NONE',  ( 44.99999999999998579, 10.00000000000000000, -57.99999999999998579 ) ) ;
#24867=ORIENTED_EDGE ( 'NONE', *, *, #26348, .F. ) ;
#24871=ORIENTED_EDGE ( 'NONE', *, *, #22772, .T. ) ;
#24889=DIRECTION ( 'NONE',  ( 0.000000000000000000, 0.000000000000000000, 1.000000000000000000 ) ) ;
#24914=ORIENTED_EDGE ( 'NONE', *, *, #28732, .F. ) ;
#24920=LINE ( 'NONE', #37879, #34034 ) ;
#24925=LINE ( 'NONE', #8536, #40087 ) ;
#24935=EDGE_LOOP ( 'NONE', ( #17788, #33909, #31615, #39028, #28236, #33428, #740, #18783, #41534, #3402, #25458, #39981, #18694, #14339, #39124, #1223 ) ) ;
#24968=DIRECTION ( 'NONE',  ( 0.000000000000000000, -0.000000000000000000, -1.000000000000000000 ) ) ;
#24973=DIRECTION ( 'NONE',  ( 0.000000000000000000, 0.000000000000000000, 1.000000000000000000 ) ) ;
#25024=ORIENTED_EDGE ( 'NONE', *, *, #33232, .T. ) ;
#25032=DIRECTION ( 'NONE',  ( 0.000000000000000000, 0.000000000000000000, 1.000000000000000000 ) ) ;
#25062=ORIENTED_EDGE ( 'NONE', *, *, #16590, .F. ) ;
#25066=CARTESIAN_POINT ( 'NONE',  ( -52.00000000000002842, -2.499999999999999556, 60.00000000000002132 ) ) ;
#25116=ORIENTED_EDGE ( 'NONE', *, *, #36416, .T. ) ;
#25119=ORIENTED_EDGE ( 'NONE', *, *, #795, .F. ) ;
#25143=ORIENTED_EDGE ( 'NONE', *, *, #16347, .T. ) ;
#25177=EDGE_CURVE ( 'NONE', #40068, #5569, #3393, .T. ) ;
#25268=ORIENTED_EDGE ( 'NONE', *, *, #9825, .T. ) ;
#25311=VECTOR ( 'NONE', #38586, 1000.000000000000000 ) ;
#25317=VECTOR ( 'NONE', #16016, 1000.000000000000000 ) ;
#25348=DIRECTION ( 'NONE',  ( 1.000000000000000000, -0.000000000000000000, -1.067522139062650178E-16 ) ) ;
#25370=DIRECTION ( 'NONE',  ( -1.000000000000000000, 0.000000000000000000, 0.000000000000000000 ) ) ;
#25387=DIRECTION ( 'NONE',  ( 1.000000000000000000, -0.000000000000000000, -0.000000000000000000 ) ) ;
#25402=CARTESIAN_POINT ( 'NONE',  ( 10.00000000000000178, 25.00000000000000000, -87.20294101747086302 ) ) ;
#25406=CIRCLE ( 'NONE', #15200, 4.000000000000003553 ) ;
#25410=EDGE_CURVE ( 'NONE', #40514, #6804, #12072, .T. ) ;
#25411=LINE ( 'NONE', #6467, #1449 ) ;
#25421=CIRCLE ( 'NONE', #15255, 10.00000000000000178 ) ;
#25444=EDGE_LOOP ( 'NONE', ( #40604, #14980, #14564, #19529 ) ) ;
#25452=ORIENTED_EDGE ( 'NONE', *, *, #32978, .T. ) ;
#25458=ORIENTED_EDGE ( 'NONE', *, *, #15723, .F. ) ;
#25463=EDGE_CURVE ( 'NONE', #31041, #31393, #31225, .T. ) ;
#25470=CIRCLE ( 'NONE', #9869, 4.000000000000003553 ) ;
#25504=VERTEX_POINT ( 'NONE', #25066 ) ;
#25528=LINE ( 'NONE', #5531, #40949 ) ;
#25543=VERTEX_POINT ( 'NONE', #11867 ) ;
#25550=ORIENTED_EDGE ( 'NONE', *, *, #18544, .T. ) ;
#25558=LINE ( 'NONE', #12362, #20806 ) ;
#25562=DIRECTION ( 'NONE',  ( 1.000000000000000000, 0.000000000000000000, 0.000000000000000000 ) ) ;
#25580=DIRECTION ( 'NONE',  ( 0.000000000000000000, 0.000000000000000000, -1.000000000000000000 ) ) ;
#25583=FACE_OUTER_BOUND ( 'NONE', #14773, .T. ) ;
#25605=DIRECTION ( 'NONE',  ( 0.000000000000000000, 0.000000000000000000, -1.000000000000000000 ) ) ;
#25626=CARTESIAN_POINT ( 'NONE',  ( -49.99999999999998579, -2.499999999999999556, 55.00000000000002132 ) ) ;
#25642=ORIENTED_EDGE ( 'NONE', *, *, #39460, .F. ) ;
#25644=EDGE_CURVE ( 'NONE', #10050, #13206, #34212, .T. ) ;
#25665=EDGE_CURVE ( 'NONE', #30811, #27676, #5490, .T. ) ;
#25712=ORIENTED_EDGE ( 'NONE', *, *, #15630, .T. ) ;
#25714=EDGE_CURVE ( 'NONE', #3291, #29490, #26118, .T. ) ;
#25736=EDGE_CURVE ( 'NONE', #28773, #38083, #18885, .T. ) ;
#25760=EDGE_CURVE ( 'NONE', #5294, #40353, #27841, .T. ) ;
#25761=VERTEX_POINT ( 'NONE', #9101 ) ;
#25809=ORIENTED_EDGE ( 'NONE', *, *, #28765, .F. ) ;
#25822=DIRECTION ( 'NONE',  ( 1.000000000000000000, -0.000000000000000000, -0.000000000000000000 ) ) ;
#25846=VECTOR ( 'NONE', #35458, 1000.000000000000000 ) ;
#25887=DIRECTION ( 'NONE',  ( 1.000000000000000000, -0.000000000000000000, -1.067522139062650178E-16 ) ) ;
#25904=LINE ( 'NONE', #13344, #9109 ) ;
#25917=VERTEX_POINT ( 'NONE', #6959 ) ;
#25922=ORIENTED_EDGE ( 'NONE', *, *, #40975, .F. ) ;
#25976=EDGE_LOOP ( 'NONE', ( #11944, #36843, #14681, #38198, #23218, #24492 ) ) ;
#25989=AXIS2_PLACEMENT_3D ( 'NONE', #28831, #2683, #25032 ) ;
#25999=EDGE_CURVE ( 'NONE', #22137, #14857, #4057, .T. ) ;
#26031=DIRECTION ( 'NONE',  ( -1.156482317317871232E-16, 0.000000000000000000, 1.000000000000000000 ) ) ;
#26040=DIRECTION ( 'NONE',  ( -1.000000000000000000, -0.000000000000000000, -0.000000000000000000 ) ) ;
#26068=ORIENTED_EDGE ( 'NONE', *, *, #26816, .T. ) ;
#26084=CARTESIAN_POINT ( 'NONE',  ( 44.99999999999998579, -2.499999999999999556, -54.99999999999999289 ) ) ;
#26092=ADVANCED_FACE ( 'NONE', ( #31540 ), #21552, .F. ) ;
#26104=CARTESIAN_POINT ( 'NONE',  ( 33.00000000000001421, -4.500000000000000000, 30.00000000000002842 ) ) ;
#26107=CARTESIAN_POINT ( 'NONE',  ( -48.00000000000001421, 10.00000000000000000, 60.00000000000002132 ) ) ;
#26118=LINE ( 'NONE', #15705, #22398 ) ;
#26129=ORIENTED_EDGE ( 'NONE', *, *, #19882, .T. ) ;
#26135=ORIENTED_EDGE ( 'NONE', *, *, #10198, .F. ) ;
#26147=LINE ( 'NONE', #179, #27784 ) ;
#26163=DIRECTION ( 'NONE',  ( 0.000000000000000000, 1.000000000000000000, -0.000000000000000000 ) ) ;
#26169=VERTEX_POINT ( 'NONE', #15174 ) ;
#26173=VECTOR ( 'NONE', #16731, 1000.000000000000000 ) ;
#26174=EDGE_LOOP ( 'NONE', ( #18539, #7030, #115, #693, #31036, #40969 ) ) ;
#26177=ORIENTED_EDGE ( 'NONE', *, *, #13316, .F. ) ;
#26178=ORIENTED_EDGE ( 'NONE', *, *, #17568, .T. ) ;
#26182=EDGE_CURVE ( 'NONE', #41076, #23612, #18573, .T. ) ;
#26199=CARTESIAN_POINT ( 'NONE',  ( 41.31041894511779589, -7.260293145401883308, 37.10439929419838734 ) ) ;
#26233=ORIENTED_EDGE ( 'NONE', *, *, #37937, .T. ) ;
#26256=CARTESIAN_POINT ( 'NONE',  ( -52.00000000000002842, 2.499999999999999556, 60.00000000000002132 ) ) ;
#26263=CARTESIAN_POINT ( 'NONE',  ( -45.00000000000002132, 10.00000000000000000, -55.00000000000000000 ) ) ;
#26291=EDGE_CURVE ( 'NONE', #18220, #7445, #9852, .T. ) ;
#26348=EDGE_CURVE ( 'NONE', #13206, #31041, #38711, .T. ) ;
#26391=ORIENTED_EDGE ( 'NONE', *, *, #13212, .T. ) ;
#26399=CARTESIAN_POINT ( 'NONE',  ( 41.49697443347378112, -7.322693517060508306, 37.16392700879935518 ) ) ;
#26403=CARTESIAN_POINT ( 'NONE',  ( -50.00000000000001421, 10.00000000000000000, 55.00000000000002132 ) ) ;
#26443=CARTESIAN_POINT ( 'NONE',  ( -50.00000000000001421, -4.500000000000000000, 40.00000000000002842 ) ) ;
#26445=SHAPE_REPRESENTATION_RELATIONSHIP ( 'NONE' , 'NONE' ,  #29355, #3124 ) ;
#26453=EDGE_CURVE ( 'NONE', #1179, #33276, #20378, .T. ) ;
#26478=DIRECTION ( 'NONE',  ( -1.000000000000000000, 0.000000000000000000, -0.000000000000000000 ) ) ;
#26503=DIRECTION ( 'NONE',  ( -0.000000000000000000, -1.000000000000000000, 0.000000000000000000 ) ) ;
#26509=AXIS2_PLACEMENT_3D ( 'NONE', #16941, #779, #13754 ) ;
#26528=VECTOR ( 'NONE', #1029, 1000.000000000000000 ) ;
#26536=DIRECTION ( 'NONE',  ( 0.000000000000000000, 0.000000000000000000, 1.000000000000000000 ) ) ;
#26542=VERTEX_POINT ( 'NONE', #8880 ) ;
#26543=EDGE_LOOP ( 'NONE', ( #32329, #19815, #1378, #37353 ) ) ;
#26545=CARTESIAN_POINT ( 'NONE',  ( 62.00000000000001421, 2.499999999999999556, -49.99999999999998579 ) ) ;
#26563=CYLINDRICAL_SURFACE ( 'NONE', #32896, 4.999999999999997335 ) ;
#26578=EDGE_CURVE ( 'NONE', #38231, #33064, #35039, .T. ) ;
#26584=VERTEX_POINT ( 'NONE', #31633 ) ;
#26586=DIRECTION ( 'NONE',  ( 0.000000000000000000, -1.734723475976805517E-15, -1.000000000000000000 ) ) ;
#26597=VERTEX_POINT ( 'NONE', #28857 ) ;
#26633=ORIENTED_EDGE ( 'NONE', *, *, #28198, .T. ) ;
#26634=CARTESIAN_POINT ( 'NONE',  ( -62.00000000000002842, 2.499999999999999556, 60.00000000000002132 ) ) ;
#26650=CARTESIAN_POINT ( 'NONE',  ( 40.50000000000000711, -15.00000000000000000, 36.00000000000002132 ) ) ;
#26681=AXIS2_PLACEMENT_3D ( 'NONE', #12838, #25822, #38786 ) ;
#26702=ADVANCED_FACE ( 'NONE', ( #37810 ), #5480, .T. ) ;
#26713=VECTOR ( 'NONE', #25887, 1000.000000000000000 ) ;
#26721=EDGE_CURVE ( 'NONE', #16039, #3104, #20134, .T. ) ;
#26745=CARTESIAN_POINT ( 'NONE',  ( -33.00000000000001421, -10.00000000000000000, 48.35164654424506381 ) ) ;
#26755=EDGE_LOOP ( 'NONE', ( #39787, #32077, #16294, #29569 ) ) ;
#26758=DIRECTION ( 'NONE',  ( 1.000000000000000000, -0.000000000000000000, -0.000000000000000000 ) ) ;
#26770=CARTESIAN_POINT ( 'NONE',  ( -45.00000000000002132, 2.499999999999999556, -59.99999999999999289 ) ) ;
#26772=ADVANCED_FACE ( 'NONE', ( #12915 ), #3135, .T. ) ;
#26814=AXIS2_PLACEMENT_3D ( 'NONE', #9411, #18981, #31948 ) ;
#26816=EDGE_CURVE ( 'NONE', #17279, #13352, #19707, .T. ) ;
#26859=ORIENTED_EDGE ( 'NONE', *, *, #39229, .T. ) ;
#26860=DIRECTION ( 'NONE',  ( -1.000000000000000000, -0.000000000000000000, -0.000000000000000000 ) ) ;
#26894=CARTESIAN_POINT ( 'NONE',  ( 38.13250975247725449, -8.049471121924245409, 41.85252274511549331 ) ) ;
#26914=ADVANCED_FACE ( 'NONE', ( #3537 ), #13122, .T. ) ;
#26925=CARTESIAN_POINT ( 'NONE',  ( -10.00000000000000178, 10.00000000000000000, -59.99999999999999289 ) ) ;
#26931=DIRECTION ( 'NONE',  ( 0.000000000000000000, -1.000000000000000000, 0.000000000000000000 ) ) ;
#26978=DIRECTION ( 'NONE',  ( -0.000000000000000000, 1.000000000000000000, -0.000000000000000000 ) ) ;
#26985=LINE ( 'NONE', #24217, #35906 ) ;
#27014=ORIENTED_EDGE ( 'NONE', *, *, #13316, .T. ) ;
#27022=LINE ( 'NONE', #23185, #37584 ) ;
#27104=CARTESIAN_POINT ( 'NONE',  ( 38.13552672522938991, -8.047467821229144391, 38.14379532929908834 ) ) ;
#27150=VECTOR ( 'NONE', #21240, 1000.000000000000000 ) ;
#27162=CARTESIAN_POINT ( 'NONE',  ( -62.00000000000001421, -2.499999999999999556, -60.00000000000000000 ) ) ;
#27177=EDGE_CURVE ( 'NONE', #12609, #1211, #10566, .T. ) ;
#27182=ORIENTED_EDGE ( 'NONE', *, *, #1030, .F. ) ;
#27203=LINE ( 'NONE', #1462, #13659 ) ;
#27210=ORIENTED_EDGE ( 'NONE', *, *, #16590, .T. ) ;
#27211=EDGE_CURVE ( 'NONE', #16352, #10050, #40104, .T. ) ;
#27220=CARTESIAN_POINT ( 'NONE',  ( 33.00000000000001421, -4.500000000000000000, 40.00000000000002842 ) ) ;
#27228=ORIENTED_EDGE ( 'NONE', *, *, #16859, .T. ) ;
#27233=DIRECTION ( 'NONE',  ( 1.000000000000000000, -2.312964634635743450E-16, 0.000000000000000000 ) ) ;
#27241=VECTOR ( 'NONE', #23557, 1000.000000000000000 ) ;
#27286=CIRCLE ( 'NONE', #15740, 4.999999999999997335 ) ;
#27320=DIRECTION ( 'NONE',  ( -0.000000000000000000, 1.000000000000000000, -0.000000000000000000 ) ) ;
#27321=CARTESIAN_POINT ( 'NONE',  ( 40.08930278741430442, -7.170401283558662797, 42.97870162680622030 ) ) ;
#27326=PLANE ( 'NONE',  #12840 ) ;
#27339=DIRECTION ( 'NONE',  ( 1.000000000000000000, -0.000000000000000000, -1.067522139062650178E-16 ) ) ;
#27361=AXIS2_PLACEMENT_3D ( 'NONE', #6706, #42037, #3718 ) ;
#27390=CIRCLE ( 'NONE', #2907, 3.000000000000016431 ) ;
#27419=ORIENTED_EDGE ( 'NONE', *, *, #16395, .F. ) ;
#27420=ADVANCED_FACE ( 'NONE', ( #3698 ), #19454, .T. ) ;
#27424=DIRECTION ( 'NONE',  ( 1.000000000000000000, -0.000000000000000000, -0.000000000000000000 ) ) ;
#27428=FACE_BOUND ( 'NONE', #6968, .T. ) ;
#27439=CARTESIAN_POINT ( 'NONE',  ( -49.99999999999998579, -2.499999999999999556, 55.00000000000002132 ) ) ;
#27440=EDGE_CURVE ( 'NONE', #25543, #41543, #27859, .T. ) ;
#27453=CARTESIAN_POINT ( 'NONE',  ( 44.99999999999998579, -10.00000000000000000, -54.99999999999999289 ) ) ;
#27480=EDGE_CURVE ( 'NONE', #14520, #26584, #9547, .T. ) ;
#27512=CARTESIAN_POINT ( 'NONE',  ( -62.00000000000001421, 2.499999999999999556, -49.99999999999998579 ) ) ;
#27527=EDGE_CURVE ( 'NONE', #33276, #20097, #35821, .T. ) ;
#27530=CARTESIAN_POINT ( 'NONE',  ( 39.69760396919353695, -7.258130416459594336, 37.10236750471068490 ) ) ;
#27538=CIRCLE ( 'NONE', #36363, 4.000000000000003553 ) ;
#27545=VERTEX_POINT ( 'NONE', #16478 ) ;
#27553=CARTESIAN_POINT ( 'NONE',  ( 44.99999999999998579, -10.00000000000000000, -57.99999999999999289 ) ) ;
#27562=CYLINDRICAL_SURFACE ( 'NONE', #41114, 4.999999999999997335 ) ;
#27592=VERTEX_POINT ( 'NONE', #28808 ) ;
#27620=VERTEX_POINT ( 'NONE', #12659 ) ;
#27649=DIRECTION ( 'NONE',  ( 0.000000000000000000, 0.000000000000000000, -1.000000000000000000 ) ) ;
#27654=FACE_OUTER_BOUND ( 'NONE', #35412, .T. ) ;
#27676=VERTEX_POINT ( 'NONE', #13908 ) ;
#27680=VERTEX_POINT ( 'NONE', #4548 ) ;
#27683=CARTESIAN_POINT ( 'NONE',  ( 40.50000000000000711, -7.145751311064572064, 43.00000000000004263 ) ) ;
#27731=FACE_OUTER_BOUND ( 'NONE', #29993, .T. ) ;
#27752=CARTESIAN_POINT ( 'NONE',  ( 52.00000000000002132, 10.00000000000000000, -49.99999999999998579 ) ) ;
#27765=FACE_OUTER_BOUND ( 'NONE', #10469, .T. ) ;
#27773=VERTEX_POINT ( 'NONE', #20504 ) ;
#27784=VECTOR ( 'NONE', #23148, 1000.000000000000000 ) ;
#27824=ORIENTED_EDGE ( 'NONE', *, *, #6965, .F. ) ;
#27829=CARTESIAN_POINT ( 'NONE',  ( 0.000000000000000000, 8.000000000000000000, 58.00000000000001421 ) ) ;
#27841=CIRCLE ( 'NONE', #7470, 10.00000000000000178 ) ;
#27859=CIRCLE ( 'NONE', #6796, 4.999999999999984013 ) ;
#27896=LINE ( 'NONE', #34906, #14006 ) ;
#27899=ORIENTED_EDGE ( 'NONE', *, *, #11391, .F. ) ;
#27920=DIRECTION ( 'NONE',  ( 0.000000000000000000, 0.000000000000000000, -1.000000000000000000 ) ) ;
#27929=ADVANCED_FACE ( 'NONE', ( #11969 ), #8573, .T. ) ;
#27942=ORIENTED_EDGE ( 'NONE', *, *, #20420, .F. ) ;
#27986=AXIS2_PLACEMENT_3D ( 'NONE', #39595, #29816, #13654 ) ;
#27990=ORIENTED_EDGE ( 'NONE', *, *, #23156, .T. ) ;
#28031=EDGE_LOOP ( 'NONE', ( #17862, #30086, #5968, #1363 ) ) ;
#28098=LINE ( 'NONE', #31289, #9551 ) ;
#28106=VECTOR ( 'NONE', #35220, 1000.000000000000000 ) ;
#28127=CIRCLE ( 'NONE', #9808, 4.999999999999997335 ) ;
#28135=DIRECTION ( 'NONE',  ( 0.000000000000000000, -1.000000000000000000, 0.000000000000000000 ) ) ;
#28142=DIRECTION ( 'NONE',  ( -1.000000000000000000, 0.000000000000000000, 0.000000000000000000 ) ) ;
#28151=ORIENTED_EDGE ( 'NONE', *, *, #9022, .T. ) ;
#28156=VECTOR ( 'NONE', #3821, 1000.000000000000000 ) ;
#28173=FACE_OUTER_BOUND ( 'NONE', #13146, .T. ) ;
#28191=DIRECTION ( 'NONE',  ( 1.156482317317871232E-16, 0.000000000000000000, 1.000000000000000000 ) ) ;
#28197=( GEOMETRIC_REPRESENTATION_CONTEXT ( 3 ) GLOBAL_UNCERTAINTY_ASSIGNED_CONTEXT ( ( #29257 ) ) GLOBAL_UNIT_ASSIGNED_CONTEXT ( ( #7086, #23686, #10916 ) ) REPRESENTATION_CONTEXT ( 'NONE', 'WORKASPACE' ) );
#28198=EDGE_CURVE ( 'NONE', #26584, #25543, #38759, .T. ) ;
#28201=AXIS2_PLACEMENT_3D ( 'NONE', #1862, #8874, #18449 ) ;
#28233=DIRECTION ( 'NONE',  ( 1.000000000000000000, 0.000000000000000000, 0.000000000000000000 ) ) ;
#28236=ORIENTED_EDGE ( 'NONE', *, *, #29300, .T. ) ;
#28251=DIRECTION ( 'NONE',  ( 0.000000000000000000, 0.000000000000000000, -1.000000000000000000 ) ) ;
#28266=EDGE_LOOP ( 'NONE', ( #25143, #39875, #30937, #15457 ) ) ;
#28289=DIRECTION ( 'NONE',  ( 0.000000000000000000, 0.000000000000000000, -1.000000000000000000 ) ) ;
#28315=DIRECTION ( 'NONE',  ( -0.000000000000000000, 1.000000000000000000, -0.000000000000000000 ) ) ;
#28335=CARTESIAN_POINT ( 'NONE',  ( -33.00000000000001421, 7.999999999999996447, 50.00000000000002842 ) ) ;
#28362=EDGE_CURVE ( 'NONE', #6804, #31075, #21793, .T. ) ;
#28368=CYLINDRICAL_SURFACE ( 'NONE', #36160, 4.999999999999997335 ) ;
#28371=DIRECTION ( 'NONE',  ( 0.000000000000000000, -1.000000000000000000, 0.000000000000000000 ) ) ;
#28374=FACE_OUTER_BOUND ( 'NONE', #16561, .T. ) ;
#28396=ORIENTED_EDGE ( 'NONE', *, *, #23242, .T. ) ;
#28405=PLANE ( 'NONE',  #18271 ) ;
#28407=ORIENTED_EDGE ( 'NONE', *, *, #2034, .F. ) ;
#28431=DIRECTION ( 'NONE',  ( 0.000000000000000000, -1.000000000000000000, 0.000000000000000000 ) ) ;
#28441=CARTESIAN_POINT ( 'NONE',  ( -73.31370849898480913, -4.500000000000000000, 40.00000000000002842 ) ) ;
#28458=EDGE_CURVE ( 'NONE', #12880, #27676, #17705, .T. ) ;
#28464=ORIENTED_EDGE ( 'NONE', *, *, #11, .F. ) ;
#28495=ORIENTED_EDGE ( 'NONE', *, *, #24646, .T. ) ;
#28530=EDGE_CURVE ( 'NONE', #18848, #25917, #32280, .T. ) ;
#28553=CARTESIAN_POINT ( 'NONE',  ( 0.000000000000000000, 10.00000000000000000, 0.000000000000000000 ) ) ;
#28564=AXIS2_PLACEMENT_3D ( 'NONE', #34518, #28135, #30920 ) ;
#28576=CARTESIAN_POINT ( 'NONE',  ( -62.00000000000002842, -2.499999999999999556, 60.00000000000002132 ) ) ;
#28599=DIRECTION ( 'NONE',  ( 0.000000000000000000, -1.000000000000000000, 0.000000000000000000 ) ) ;
#28606=ORIENTED_EDGE ( 'NONE', *, *, #32513, .T. ) ;
#28659=DIRECTION ( 'NONE',  ( -0.000000000000000000, 1.000000000000000000, -0.000000000000000000 ) ) ;
#28664=CIRCLE ( 'NONE', #21869, 4.000000000000003553 ) ;
#28673=AXIS2_PLACEMENT_3D ( 'NONE', #10165, #806, #16149 ) ;
#28674=CIRCLE ( 'NONE', #13718, 3.000000000000002665 ) ;
#28713=EDGE_CURVE ( 'NONE', #4822, #40068, #31293, .T. ) ;
#28732=EDGE_CURVE ( 'NONE', #25761, #23938, #39075, .T. ) ;
#28747=FACE_OUTER_BOUND ( 'NONE', #28031, .T. ) ;
#28757=ORIENTED_EDGE ( 'NONE', *, *, #38610, .F. ) ;
#28765=EDGE_CURVE ( 'NONE', #13352, #25761, #19735, .T. ) ;
#28773=VERTEX_POINT ( 'NONE', #3973 ) ;
#28782=DIRECTION ( 'NONE',  ( 0.000000000000000000, -1.000000000000000000, 0.000000000000000000 ) ) ;
#28783=VECTOR ( 'NONE', #39267, 1000.000000000000000 ) ;
#28808=CARTESIAN_POINT ( 'NONE',  ( -50.00000000000001421, 2.499999999999999556, 55.00000000000002132 ) ) ;
#28821=DIRECTION ( 'NONE',  ( 0.000000000000000000, 0.000000000000000000, -1.000000000000000000 ) ) ;
#28830=EDGE_LOOP ( 'NONE', ( #9711, #10839 ) ) ;
#28831=CARTESIAN_POINT ( 'NONE',  ( 47.99999999999998579, 10.00000000000000000, 60.00000000000002132 ) ) ;
#28833=CARTESIAN_POINT ( 'NONE',  ( -33.00000000000001421, -4.500000000000000888, 50.00000000000002842 ) ) ;
#28857=CARTESIAN_POINT ( 'NONE',  ( 49.99999999999998579, -2.499999999999999556, 36.53589838486225005 ) ) ;
#28865=ORIENTED_EDGE ( 'NONE', *, *, #8933, .T. ) ;
#28870=PLANE ( 'NONE',  #41040 ) ;
#28880=VERTEX_POINT ( 'NONE', #30764 ) ;
#28892=AXIS2_PLACEMENT_3D ( 'NONE', #26107, #32679, #3541 ) ;
#28933=ORIENTED_EDGE ( 'NONE', *, *, #20770, .T. ) ;
#28941=ORIENTED_EDGE ( 'NONE', *, *, #40942, .T. ) ;
#28961=PLANE ( 'NONE',  #26814 ) ;
#28971=DIRECTION ( 'NONE',  ( 0.000000000000000000, 0.000000000000000000, 1.000000000000000000 ) ) ;
#28972=CARTESIAN_POINT ( 'NONE',  ( -48.00000000000001421, 8.000000000000000000, -54.99999999999997158 ) ) ;
#29037=EDGE_LOOP ( 'NONE', ( #31390, #37880, #2794, #25550 ) ) ;
#29039=FACE_OUTER_BOUND ( 'NONE', #11117, .T. ) ;
#29052=ADVANCED_FACE ( 'NONE', ( #38183 ), #2878, .F. ) ;
#29066=CARTESIAN_POINT ( 'NONE',  ( -33.00000000000001421, -4.500000000000000000, 40.00000000000002842 ) ) ;
#29139=ORIENTED_EDGE ( 'NONE', *, *, #26721, .T. ) ;
#29222=CARTESIAN_POINT ( 'NONE',  ( 0.000000000000000000, 10.00000000000000000, 0.000000000000000000 ) ) ;
#29257=UNCERTAINTY_MEASURE_WITH_UNIT (LENGTH_MEASURE( 1.000000000000000082E-05 ), #7086, 'distance_accuracy_value', 'NONE');
#29259=LINE ( 'NONE', #6527, #327 ) ;
#29267=CARTESIAN_POINT ( 'NONE',  ( -33.00000000000001421, -4.500000000000000888, 50.00000000000002842 ) ) ;
#29270=FACE_OUTER_BOUND ( 'NONE', #16817, .T. ) ;
#29277=EDGE_CURVE ( 'NONE', #6615, #8493, #40582, .T. ) ;
#29279=DIRECTION ( 'NONE',  ( 1.000000000000000000, 0.000000000000000000, 0.000000000000000000 ) ) ;
#29281=CARTESIAN_POINT ( 'NONE',  ( 44.99999999999998579, 10.00000000000000000, 60.00000000000002132 ) ) ;
#29282=CARTESIAN_POINT ( 'NONE',  ( 38.98014376739327247, -7.548381381975341142, 42.59332567428268845 ) ) ;
#29300=EDGE_CURVE ( 'NONE', #13199, #27545, #27203, .T. ) ;
#29317=CARTESIAN_POINT ( 'NONE',  ( 49.99999999999998579, 2.499999999999999556, -54.99999999999997158 ) ) ;
#29325=FACE_OUTER_BOUND ( 'NONE', #2715, .T. ) ;
#29331=CARTESIAN_POINT ( 'NONE',  ( -45.00000000000002132, -10.00000000000000000, -59.99999999999999289 ) ) ;
#29339=CIRCLE ( 'NONE', #34789, 4.999999999999984013 ) ;
#29341=EDGE_LOOP ( 'NONE', ( #32581, #21086, #39606, #27824 ) ) ;
#29345=DIRECTION ( 'NONE',  ( 1.000000000000000000, -0.000000000000000000, -0.000000000000000000 ) ) ;
#29349=ORIENTED_EDGE ( 'NONE', *, *, #15480, .F. ) ;
#29353=ORIENTED_EDGE ( 'NONE', *, *, #32513, .F. ) ;
#29355=SHAPE_REPRESENTATION ( 'Main Plastic Part', ( #40442 ), #28197 ) ;
#29356=AXIS2_PLACEMENT_3D ( 'NONE', #3019, #16011, #30 ) ;
#29362=CARTESIAN_POINT ( 'NONE',  ( 43.50040773475621592, -8.500305800795507238, 39.79993359057041857 ) ) ;
#29377=CARTESIAN_POINT ( 'NONE',  ( -50.00000000000001421, 10.00000000000000000, -55.00000000000000000 ) ) ;
#29381=ORIENTED_EDGE ( 'NONE', *, *, #26291, .F. ) ;
#29383=CARTESIAN_POINT ( 'NONE',  ( -10.00000000000000178, 10.00000000000000000, -87.20294101747086302 ) ) ;
#29406=EDGE_CURVE ( 'NONE', #24557, #6615, #24540, .T. ) ;
#29408=DIRECTION ( 'NONE',  ( 0.000000000000000000, 0.000000000000000000, -1.000000000000000000 ) ) ;
#29415=CARTESIAN_POINT ( 'NONE',  ( -45.00000000000002132, 10.00000000000000000, -55.00000000000000000 ) ) ;
#29429=AXIS2_PLACEMENT_3D ( 'NONE', #15709, #18470, #31437 ) ;
#29446=VERTEX_POINT ( 'NONE', #1986 ) ;
#29475=DIRECTION ( 'NONE',  ( 0.000000000000000000, -1.000000000000000000, 0.000000000000000000 ) ) ;
#29482=DIRECTION ( 'NONE',  ( 0.000000000000000000, 1.000000000000000000, -5.551115123125782702E-16 ) ) ;
#29483=DIRECTION ( 'NONE',  ( -0.000000000000000000, -1.000000000000000000, -0.000000000000000000 ) ) ;
#29490=VERTEX_POINT ( 'NONE', #11764 ) ;
#29497=CARTESIAN_POINT ( 'NONE',  ( -33.00000000000001421, -4.500000000000000000, 40.00000000000002842 ) ) ;
#29509=CARTESIAN_POINT ( 'NONE',  ( 40.50000000000000711, -10.00000000000000000, 36.00000000000002132 ) ) ;
#29569=ORIENTED_EDGE ( 'NONE', *, *, #33336, .F. ) ;
#29572=EDGE_LOOP ( 'NONE', ( #9522, #40658, #35948, #31873 ) ) ;
#29579=CARTESIAN_POINT ( 'NONE',  ( 41.49594703006624741, -7.322379418330077883, 42.83635789519335901 ) ) ;
#29720=ORIENTED_EDGE ( 'NONE', *, *, #1030, .T. ) ;
#29725=ORIENTED_EDGE ( 'NONE', *, *, #23011, .T. ) ;
#29729=ORIENTED_EDGE ( 'NONE', *, *, #9381, .T. ) ;
#29740=CARTESIAN_POINT ( 'NONE',  ( 44.99999999999999289, 10.00000000000000000, 55.00000000000002132 ) ) ;
#29762=ORIENTED_EDGE ( 'NONE', *, *, #29300, .F. ) ;
#29766=ORIENTED_EDGE ( 'NONE', *, *, #12828, .T. ) ;
#29789=CARTESIAN_POINT ( 'NONE',  ( 41.85224782803753385, -7.466852685707067394, 37.31509891355641884 ) ) ;
#29813=CARTESIAN_POINT ( 'NONE',  ( 47.99999999999998579, -10.00000000000000000, 0.000000000000000000 ) ) ;
#29816=DIRECTION ( 'NONE',  ( 1.000000000000000000, -0.000000000000000000, -0.000000000000000000 ) ) ;
#29822=DIRECTION ( 'NONE',  ( 0.000000000000000000, 0.000000000000000000, 1.000000000000000000 ) ) ;
#29843=CARTESIAN_POINT ( 'NONE',  ( -48.00000000000002132, -10.00000000000000000, -54.99999999999998579 ) ) ;
#29865=CARTESIAN_POINT ( 'NONE',  ( 11.00000000000000355, 10.00000000000000000, 60.00000000000002132 ) ) ;
#29916=CARTESIAN_POINT ( 'NONE',  ( 49.99999999999998579, 10.00000000000000000, -54.99999999999997158 ) ) ;
#29923=DIRECTION ( 'NONE',  ( 0.000000000000000000, 0.000000000000000000, -1.000000000000000000 ) ) ;
#29934=PLANE ( 'NONE',  #28673 ) ;
#29983=EDGE_CURVE ( 'NONE', #12609, #33064, #11508, .T. ) ;
#29985=DIRECTION ( 'NONE',  ( 2.312964634635743450E-16, 1.000000000000000000, 0.000000000000000000 ) ) ;
#29993=EDGE_LOOP ( 'NONE', ( #41744, #6133, #30140, #5259 ) ) ;
#30067=EDGE_CURVE ( 'NONE', #36692, #16441, #24920, .T. ) ;
#30080=AXIS2_PLACEMENT_3D ( 'NONE', #36151, #27233, #29985 ) ;
#30084=EDGE_LOOP ( 'NONE', ( #37367, #18689, #32426, #26633 ) ) ;
#30086=ORIENTED_EDGE ( 'NONE', *, *, #26816, .F. ) ;
#30140=ORIENTED_EDGE ( 'NONE', *, *, #20955, .F. ) ;
#30141=ORIENTED_EDGE ( 'NONE', *, *, #35447, .T. ) ;
#30146=VERTEX_POINT ( 'NONE', #2990 ) ;
#30152=AXIS2_PLACEMENT_3D ( 'NONE', #31066, #30651, #14898 ) ;
#30167=DIRECTION ( 'NONE',  ( 0.000000000000000000, 0.000000000000000000, -1.000000000000000000 ) ) ;
#30176=PLANE ( 'NONE',  #8689 ) ;
#30196=ORIENTED_EDGE ( 'NONE', *, *, #40439, .T. ) ;
#30204=ORIENTED_EDGE ( 'NONE', *, *, #8544, .T. ) ;
#30229=LINE ( 'NONE', #10038, #2971 ) ;
#30254=DIRECTION ( 'NONE',  ( -0.000000000000000000, 1.000000000000000000, -0.000000000000000000 ) ) ;
#30289=CARTESIAN_POINT ( 'NONE',  ( 37.50043185558879344, -8.499676108608733571, 39.78792392633494757 ) ) ;
#30309=EDGE_CURVE ( 'NONE', #20613, #35430, #10079, .T. ) ;
#30320=CARTESIAN_POINT ( 'NONE',  ( -45.00000000000002132, -10.00000000000000000, -57.99999999999998579 ) ) ;
#30337=CARTESIAN_POINT ( 'NONE',  ( 40.50000000000000711, -15.00000000000000000, 40.00000000000002842 ) ) ;
#30344=LINE ( 'NONE', #1217, #30710 ) ;
#30359=ORIENTED_EDGE ( 'NONE', *, *, #14472, .F. ) ;
#30360=DIRECTION ( 'NONE',  ( 0.000000000000000000, 0.000000000000000000, -1.000000000000000000 ) ) ;
#30364=EDGE_CURVE ( 'NONE', #15972, #746, #11761, .T. ) ;
#30497=CARTESIAN_POINT ( 'NONE',  ( 37.49958095599880892, -8.500314282705053515, 40.19967692501300860 ) ) ;
#30522=ADVANCED_FACE ( 'NONE', ( #18156 ), #31127, .T. ) ;
#30532=CARTESIAN_POINT ( 'NONE',  ( 49.99999999999998579, 10.00000000000000000, 55.00000000000002132 ) ) ;
#30534=LINE ( 'NONE', #15214, #7714 ) ;
#30569=ORIENTED_EDGE ( 'NONE', *, *, #8224, .F. ) ;
#30584=VECTOR ( 'NONE', #32590, 1000.000000000000000 ) ;
#30600=CARTESIAN_POINT ( 'NONE',  ( 47.99999999999998579, 8.000000000000000000, 50.00000000000002842 ) ) ;
#30621=LINE ( 'NONE', #27439, #35522 ) ;
#30630=ADVANCED_FACE ( 'NONE', ( #18786 ), #2410, .T. ) ;
#30651=DIRECTION ( 'NONE',  ( -0.000000000000000000, 1.000000000000000000, -0.000000000000000000 ) ) ;
#30657=CARTESIAN_POINT ( 'NONE',  ( 0.000000000000000000, 8.000000000000000000, -57.99999999999998579 ) ) ;
#30675=AXIS2_PLACEMENT_3D ( 'NONE', #15103, #21683, #5523 ) ;
#30710=VECTOR ( 'NONE', #20787, 1000.000000000000000 ) ;
#30714=CARTESIAN_POINT ( 'NONE',  ( 37.66389073306345381, -8.378221026928336812, 40.99790684889472203 ) ) ;
#30723=AXIS2_PLACEMENT_3D ( 'NONE', #27220, #1273, #4869 ) ;
#30728=CARTESIAN_POINT ( 'NONE',  ( 44.99999999999999289, -2.499999999999999556, 55.00000000000002132 ) ) ;
#30731=EDGE_LOOP ( 'NONE', ( #13714, #12244, #9590, #5227 ) ) ;
#30755=VECTOR ( 'NONE', #112, 1000.000000000000000 ) ;
#30764=CARTESIAN_POINT ( 'NONE',  ( 33.00000000000001421, -10.00000000000000000, 48.35164654424506381 ) ) ;
#30786=AXIS2_PLACEMENT_3D ( 'NONE', #10906, #26860, #20479 ) ;
#30811=VERTEX_POINT ( 'NONE', #20040 ) ;
#30814=AXIS2_PLACEMENT_3D ( 'NONE', #30337, #1210, #11970 ) ;
#30824=ORIENTED_EDGE ( 'NONE', *, *, #10263, .T. ) ;
#30828=ORIENTED_EDGE ( 'NONE', *, *, #1489, .T. ) ;
#30865=CARTESIAN_POINT ( 'NONE',  ( -45.00000000000002132, 10.00000000000000000, -57.99999999999998579 ) ) ;
#30914=VECTOR ( 'NONE', #13744, 1000.000000000000000 ) ;
#30920=DIRECTION ( 'NONE',  ( 0.000000000000000000, 0.000000000000000000, -1.000000000000000000 ) ) ;
#30937=ORIENTED_EDGE ( 'NONE', *, *, #17113, .F. ) ;
#30994=EDGE_CURVE ( 'NONE', #26542, #14857, #2306, .T. ) ;
#31032=LINE ( 'NONE', #18475, #9001 ) ;
#31036=ORIENTED_EDGE ( 'NONE', *, *, #6159, .T. ) ;
#31040=LINE ( 'NONE', #15089, #11083 ) ;
#31041=VERTEX_POINT ( 'NONE', #33854 ) ;
#31066=CARTESIAN_POINT ( 'NONE',  ( -45.00000000000002132, 10.00000000000000000, 55.00000000000002132 ) ) ;
#31075=VERTEX_POINT ( 'NONE', #14087 ) ;
#31083=ORIENTED_EDGE ( 'NONE', *, *, #15512, .T. ) ;
#31114=DIRECTION ( 'NONE',  ( 0.000000000000000000, 1.000000000000000000, -0.000000000000000000 ) ) ;
#31126=CARTESIAN_POINT ( 'NONE',  ( 49.99999999999998579, 10.00000000000000000, -55.00000000000000000 ) ) ;
#31127=PLANE ( 'NONE',  #34548 ) ;
#31128=PLANE ( 'NONE',  #6946 ) ;
#31140=EDGE_LOOP ( 'NONE', ( #32962, #24871, #15049, #7607, #41891, #21828 ) ) ;
#31159=DIRECTION ( 'NONE',  ( -0.000000000000000000, -1.000000000000000000, -0.000000000000000000 ) ) ;
#31185=ORIENTED_EDGE ( 'NONE', *, *, #24646, .F. ) ;
#31195=ORIENTED_EDGE ( 'NONE', *, *, #11873, .F. ) ;
#31206=AXIS2_PLACEMENT_3D ( 'NONE', #21247, #24241, #28251 ) ;
#31225=LINE ( 'NONE', #2087, #27150 ) ;
#31244=AXIS2_PLACEMENT_3D ( 'NONE', #38095, #21513, #8328 ) ;
#31286=ORIENTED_EDGE ( 'NONE', *, *, #2034, .T. ) ;
#31287=EDGE_CURVE ( 'NONE', #38083, #27680, #42036, .T. ) ;
#31289=CARTESIAN_POINT ( 'NONE',  ( -48.00000000000001421, -4.500000000000000000, 30.00000000000002842 ) ) ;
#31292=VERTEX_POINT ( 'NONE', #12294 ) ;
#31293=CIRCLE ( 'NONE', #4121, 3.000000000000002665 ) ;
#31322=CARTESIAN_POINT ( 'NONE',  ( 33.00000000000001421, -4.500000000000000888, 50.00000000000002842 ) ) ;
#31385=VECTOR ( 'NONE', #21451, 1000.000000000000000 ) ;
#31390=ORIENTED_EDGE ( 'NONE', *, *, #26348, .T. ) ;
#31393=VERTEX_POINT ( 'NONE', #7386 ) ;
#31418=CARTESIAN_POINT ( 'NONE',  ( 44.99999999999999289, 10.00000000000000000, 55.00000000000002132 ) ) ;
#31437=DIRECTION ( 'NONE',  ( 0.000000000000000000, 0.000000000000000000, -1.000000000000000000 ) ) ;
#31457=ORIENTED_EDGE ( 'NONE', *, *, #21158, .F. ) ;
#31463=VECTOR ( 'NONE', #29475, 1000.000000000000000 ) ;
#31467=AXIS2_PLACEMENT_3D ( 'NONE', #23344, #12724, #39080 ) ;
#31495=DIRECTION ( 'NONE',  ( -1.156482317317871232E-16, -0.000000000000000000, -1.000000000000000000 ) ) ;
#31499=CARTESIAN_POINT ( 'NONE',  ( 62.00000000000001421, -2.499999999999999556, -49.99999999999998579 ) ) ;
#31505=DIRECTION ( 'NONE',  ( 0.000000000000000000, -1.000000000000000000, 0.000000000000000000 ) ) ;
#31509=LINE ( 'NONE', #34286, #22731 ) ;
#31540=FACE_OUTER_BOUND ( 'NONE', #5510, .T. ) ;
#31541=VECTOR ( 'NONE', #33095, 1000.000000000000000 ) ;
#31551=EDGE_CURVE ( 'NONE', #27592, #6074, #39497, .T. ) ;
#31581=LINE ( 'NONE', #31782, #23243 ) ;
#31593=DIRECTION ( 'NONE',  ( -1.000000000000000000, 0.000000000000000000, 1.156482317317871232E-16 ) ) ;
#31614=CARTESIAN_POINT ( 'NONE',  ( 40.50000000000000711, 10.00099999999999945, 40.00000000000002842 ) ) ;
#31615=ORIENTED_EDGE ( 'NONE', *, *, #17810, .T. ) ;
#31627=LINE ( 'NONE', #41420, #21402 ) ;
#31628=LINE ( 'NONE', #21224, #36813 ) ;
#31633=CARTESIAN_POINT ( 'NONE',  ( -50.00000000000001421, 10.00000000000000000, -54.99999999999997158 ) ) ;
#31638=DIRECTION ( 'NONE',  ( 0.000000000000000000, 0.000000000000000000, 1.000000000000000000 ) ) ;
#31648=FACE_OUTER_BOUND ( 'NONE', #33218, .T. ) ;
#31651=ORIENTED_EDGE ( 'NONE', *, *, #14132, .T. ) ;
#31653=ADVANCED_FACE ( 'NONE', ( #19468 ), #28405, .F. ) ;
#31661=CARTESIAN_POINT ( 'NONE',  ( 44.99999999999999289, 2.499999999999999556, 55.00000000000002132 ) ) ;
#31662=CYLINDRICAL_SURFACE ( 'NONE', #34968, 4.000000000000003553 ) ;
#31681=EDGE_CURVE ( 'NONE', #5569, #32443, #20309, .T. ) ;
#31701=ORIENTED_EDGE ( 'NONE', *, *, #30994, .F. ) ;
#31731=PLANE ( 'NONE',  #22098 ) ;
#31733=ORIENTED_EDGE ( 'NONE', *, *, #33398, .F. ) ;
#31757=ORIENTED_EDGE ( 'NONE', *, *, #13784, .T. ) ;
#31782=CARTESIAN_POINT ( 'NONE',  ( -45.00000000000002132, 10.00000000000000000, 58.00000000000001421 ) ) ;
#31795=CARTESIAN_POINT ( 'NONE',  ( -11.00000000000000355, 26.00000000000000355, 60.00000000000002132 ) ) ;
#31809=ADVANCED_FACE ( 'NONE', ( #19877, #1165 ), #32637, .F. ) ;
#31811=CYLINDRICAL_SURFACE ( 'NONE', #23971, 4.999999999999997335 ) ;
#31850=CARTESIAN_POINT ( 'NONE',  ( 49.99999999999998579, -2.499999999999999556, 55.00000000000002132 ) ) ;
#31852=DIRECTION ( 'NONE',  ( 0.000000000000000000, 0.000000000000000000, 1.000000000000000000 ) ) ;
#31873=ORIENTED_EDGE ( 'NONE', *, *, #37845, .F. ) ;
#31900=VECTOR ( 'NONE', #28233, 1000.000000000000000 ) ;
#31948=DIRECTION ( 'NONE',  ( 0.000000000000000000, -0.000000000000000000, -1.000000000000000000 ) ) ;
#31964=AXIS2_PLACEMENT_3D ( 'NONE', #2134, #8723, #34671 ) ;
#31972=AXIS2_PLACEMENT_3D ( 'NONE', #35853, #26503, #39889 ) ;
#31987=DIRECTION ( 'NONE',  ( 0.000000000000000000, 0.000000000000000000, -1.000000000000000000 ) ) ;
#31989=ADVANCED_FACE ( 'NONE', ( #27731 ), #27326, .T. ) ;
#32019=DIRECTION ( 'NONE',  ( -0.000000000000000000, 1.000000000000000000, -0.000000000000000000 ) ) ;
#32073=ORIENTED_EDGE ( 'NONE', *, *, #20167, .F. ) ;
#32077=ORIENTED_EDGE ( 'NONE', *, *, #25410, .F. ) ;
#32131=ADVANCED_FACE ( 'NONE', ( #37934 ), #15605, .T. ) ;
#32139=EDGE_LOOP ( 'NONE', ( #27942, #29139, #10731, #29381 ) ) ;
#32158=DIRECTION ( 'NONE',  ( 0.000000000000000000, 0.000000000000000000, 1.000000000000000000 ) ) ;
#32161=ORIENTED_EDGE ( 'NONE', *, *, #18324, .T. ) ;
#32170=ORIENTED_EDGE ( 'NONE', *, *, #4337, .F. ) ;
#32246=VECTOR ( 'NONE', #5831, 1000.000000000000000 ) ;
#32248=DIRECTION ( 'NONE',  ( -1.000000000000000000, 0.000000000000000000, 0.000000000000000000 ) ) ;
#32275=AXIS2_PLACEMENT_3D ( 'NONE', #7932, #17709, #34493 ) ;
#32280=LINE ( 'NONE', #30865, #19065 ) ;
#32281=CARTESIAN_POINT ( 'NONE',  ( -50.00000000000001421, 10.00000000000000000, 58.00000000000001421 ) ) ;
#32325=ADVANCED_FACE ( 'NONE', ( #13875 ), #20472, .T. ) ;
#32329=ORIENTED_EDGE ( 'NONE', *, *, #19882, .F. ) ;
#32367=CARTESIAN_POINT ( 'NONE',  ( 33.00000000000001421, -4.500000000000000000, 30.00000000000002842 ) ) ;
#32409=FACE_OUTER_BOUND ( 'NONE', #35423, .T. ) ;
#32420=DIRECTION ( 'NONE',  ( 0.000000000000000000, 0.000000000000000000, -1.000000000000000000 ) ) ;
#32421=EDGE_CURVE ( 'NONE', #27773, #21965, #26147, .T. ) ;
#32426=ORIENTED_EDGE ( 'NONE', *, *, #13212, .F. ) ;
#32430=PLANE ( 'NONE',  #11834 ) ;
#32436=DIRECTION ( 'NONE',  ( 0.000000000000000000, 0.000000000000000000, -1.000000000000000000 ) ) ;
#32443=VERTEX_POINT ( 'NONE', #39097 ) ;
#32474=CARTESIAN_POINT ( 'NONE',  ( 52.00000000000002842, -2.499999999999999556, 50.00000000000001421 ) ) ;
#32513=EDGE_CURVE ( 'NONE', #13040, #19396, #26985, .T. ) ;
#32530=DIRECTION ( 'NONE',  ( 1.000000000000000000, -0.000000000000000000, -0.000000000000000000 ) ) ;
#32556=CARTESIAN_POINT ( 'NONE',  ( 42.86775675088892967, -8.049649642115912940, 38.14782173530672793 ) ) ;
#32560=VECTOR ( 'NONE', #12398, 1000.000000000000000 ) ;
#32561=DIRECTION ( 'NONE',  ( -0.000000000000000000, 1.000000000000000000, -0.000000000000000000 ) ) ;
#32570=CARTESIAN_POINT ( 'NONE',  ( -10.00000000000000178, 10.00000000000000000, 60.00000000000002132 ) ) ;
#32575=ORIENTED_EDGE ( 'NONE', *, *, #26721, .F. ) ;
#32581=ORIENTED_EDGE ( 'NONE', *, *, #25760, .F. ) ;
#32590=DIRECTION ( 'NONE',  ( 0.000000000000000000, 0.000000000000000000, 1.000000000000000000 ) ) ;
#32637=PLANE ( 'NONE',  #1285 ) ;
#32650=EDGE_LOOP ( 'NONE', ( #11560, #31286, #14350, #38551 ) ) ;
#32679=DIRECTION ( 'NONE',  ( 1.000000000000000000, -0.000000000000000000, 0.000000000000000000 ) ) ;
#32683=LINE ( 'NONE', #16539, #28783 ) ;
#32688=DIRECTION ( 'NONE',  ( 0.000000000000000000, 0.000000000000000000, -1.000000000000000000 ) ) ;
#32693=PLANE ( 'NONE',  #31467 ) ;
#32703=ORIENTED_EDGE ( 'NONE', *, *, #39829, .T. ) ;
#32709=LINE ( 'NONE', #38473, #4775 ) ;
#32740=ORIENTED_EDGE ( 'NONE', *, *, #28732, .T. ) ;
#32748=DIRECTION ( 'NONE',  ( 0.000000000000000000, 1.000000000000000000, -0.000000000000000000 ) ) ;
#32762=CIRCLE ( 'NONE', #34119, 10.00000000000000178 ) ;
#32763=CARTESIAN_POINT ( 'NONE',  ( 42.74198171570055393, -7.966342543768213602, 42.00222127956244123 ) ) ;
#32782=VERTEX_POINT ( 'NONE', #12269 ) ;
#32795=CIRCLE ( 'NONE', #15826, 4.999999999999997335 ) ;
#32797=ADVANCED_FACE ( 'NONE', ( #18237 ), #5894, .F. ) ;
#32829=DIRECTION ( 'NONE',  ( -1.000000000000000000, -0.000000000000000000, -0.000000000000000000 ) ) ;
#32833=ORIENTED_EDGE ( 'NONE', *, *, #27527, .F. ) ;
#32835=CIRCLE ( 'NONE', #9073, 4.000000000000003553 ) ;
#32853=CYLINDRICAL_SURFACE ( 'NONE', #27361, 4.000000000000010658 ) ;
#32865=ADVANCED_FACE ( 'NONE', ( #5472, #15053, #18032 ), #2700, .T. ) ;
#32889=PLANE ( 'NONE',  #28892 ) ;
#32896=AXIS2_PLACEMENT_3D ( 'NONE', #29740, #13579, #30167 ) ;
#32936=CARTESIAN_POINT ( 'NONE',  ( 47.99999999999998579, 8.000000000000000000, 30.00000000000002487 ) ) ;
#32959=LINE ( 'NONE', #19776, #1517 ) ;
#32962=ORIENTED_EDGE ( 'NONE', *, *, #35925, .F. ) ;
#32973=EDGE_LOOP ( 'NONE', ( #14415, #12663, #13836, #21668 ) ) ;
#32978=EDGE_CURVE ( 'NONE', #1841, #31292, #31627, .T. ) ;
#32980=CARTESIAN_POINT ( 'NONE',  ( 43.47741575151630400, -8.482991578102483388, 40.41967448407618946 ) ) ;
#32988=LINE ( 'NONE', #9838, #17873 ) ;
#33042=ADVANCED_FACE ( 'NONE', ( #37389 ), #8246, .F. ) ;
#33064=VERTEX_POINT ( 'NONE', #39054 ) ;
#33075=CARTESIAN_POINT ( 'NONE',  ( 33.00000000000001421, -4.500000000000000000, 40.00000000000002842 ) ) ;
#33079=LINE ( 'NONE', #13516, #8208 ) ;
#33086=CARTESIAN_POINT ( 'NONE',  ( 44.99999999999998579, 10.00000000000000000, -59.99999999999999289 ) ) ;
#33095=DIRECTION ( 'NONE',  ( 0.000000000000000000, 0.000000000000000000, -1.000000000000000000 ) ) ;
#33142=DIRECTION ( 'NONE',  ( 0.000000000000000000, -0.000000000000000000, -1.000000000000000000 ) ) ;
#33144=DIRECTION ( 'NONE',  ( 1.000000000000000000, -0.000000000000000000, 0.000000000000000000 ) ) ;
#33161=CARTESIAN_POINT ( 'NONE',  ( 62.00000000000002842, 2.499999999999999556, 60.00000000000002132 ) ) ;
#33184=EDGE_CURVE ( 'NONE', #35847, #33611, #29259, .T. ) ;
#33212=LINE ( 'NONE', #29813, #19015 ) ;
#33218=EDGE_LOOP ( 'NONE', ( #24334, #28151, #11226, #5084, #28396, #28941 ) ) ;
#33232=EDGE_CURVE ( 'NONE', #27680, #8493, #37140, .T. ) ;
#33260=CARTESIAN_POINT ( 'NONE',  ( 38.66845661344590468, -7.715154313405583331, 42.38343236611764553 ) ) ;
#33276=VERTEX_POINT ( 'NONE', #33086 ) ;
#33290=FACE_OUTER_BOUND ( 'NONE', #19375, .T. ) ;
#33297=CARTESIAN_POINT ( 'NONE',  ( -48.00000000000001421, 7.999999999999996447, 50.00000000000002842 ) ) ;
#33336=EDGE_CURVE ( 'NONE', #31075, #35847, #36708, .T. ) ;
#33338=FACE_OUTER_BOUND ( 'NONE', #35749, .T. ) ;
#33373=DIRECTION ( 'NONE',  ( 0.000000000000000000, 0.000000000000000000, -1.000000000000000000 ) ) ;
#33378=ORIENTED_EDGE ( 'NONE', *, *, #17065, .F. ) ;
#33398=EDGE_CURVE ( 'NONE', #9969, #13780, #17146, .T. ) ;
#33400=VECTOR ( 'NONE', #5104, 1000.000000000000000 ) ;
#33428=ORIENTED_EDGE ( 'NONE', *, *, #10228, .T. ) ;
#33430=CARTESIAN_POINT ( 'NONE',  ( -33.00000000000001421, -10.00000000000000000, 48.35164654424506381 ) ) ;
#33431=DIRECTION ( 'NONE',  ( 1.000000000000000000, -0.000000000000000000, -1.067522139062650178E-16 ) ) ;
#33432=ORIENTED_EDGE ( 'NONE', *, *, #19885, .F. ) ;
#33440=CARTESIAN_POINT ( 'NONE',  ( 33.00000000000001421, 7.999999999999996447, 50.00000000000002842 ) ) ;
#33463=ADVANCED_FACE ( 'NONE', ( #18188 ), #27562, .T. ) ;
#33477=ORIENTED_EDGE ( 'NONE', *, *, #12455, .F. ) ;
#33480=CARTESIAN_POINT ( 'NONE',  ( 38.98408443455777928, -7.546394839972037971, 37.40433256802030826 ) ) ;
#33486=VECTOR ( 'NONE', #11936, 1000.000000000000000 ) ;
#33491=EDGE_LOOP ( 'NONE', ( #11570, #34830, #26859, #17236 ) ) ;
#33493=ORIENTED_EDGE ( 'NONE', *, *, #37619, .T. ) ;
#33518=LINE ( 'NONE', #7357, #13307 ) ;
#33551=ORIENTED_EDGE ( 'NONE', *, *, #31681, .T. ) ;
#33560=DIRECTION ( 'NONE',  ( -0.000000000000000000, -1.000000000000000000, 0.000000000000000000 ) ) ;
#33611=VERTEX_POINT ( 'NONE', #3481 ) ;
#33660=VERTEX_POINT ( 'NONE', #26256 ) ;
#33715=ORIENTED_EDGE ( 'NONE', *, *, #20770, .F. ) ;
#33737=CARTESIAN_POINT ( 'NONE',  ( 62.00000000000002842, 2.499999999999999556, 50.00000000000001421 ) ) ;
#33757=DIRECTION ( 'NONE',  ( -1.156482317317871232E-16, 0.000000000000000000, 1.000000000000000000 ) ) ;
#33774=PLANE ( 'NONE',  #34644 ) ;
#33796=DIRECTION ( 'NONE',  ( 0.000000000000000000, -1.000000000000000000, 0.000000000000000000 ) ) ;
#33806=CARTESIAN_POINT ( 'NONE',  ( -11.00000000000000355, 10.00000000000000000, -59.99999999999999289 ) ) ;
#33851=EDGE_LOOP ( 'NONE', ( #18152, #7974 ) ) ;
#33854=CARTESIAN_POINT ( 'NONE',  ( 47.99999999999998579, 8.000000000000000000, 55.00000000000002132 ) ) ;
#33902=CARTESIAN_POINT ( 'NONE',  ( 39.50698976456946809, -7.321305292375414275, 37.16256626052705769 ) ) ;
#33909=ORIENTED_EDGE ( 'NONE', *, *, #40363, .T. ) ;
#33915=CIRCLE ( 'NONE', #6737, 4.000000000000003553 ) ;
#33921=ORIENTED_EDGE ( 'NONE', *, *, #795, .T. ) ;
#33924=DIRECTION ( 'NONE',  ( 0.000000000000000000, -1.000000000000000000, 0.000000000000000000 ) ) ;
#33971=ORIENTED_EDGE ( 'NONE', *, *, #14944, .F. ) ;
#33972=PLANE ( 'NONE',  #6247 ) ;
#34025=EDGE_CURVE ( 'NONE', #9431, #32782, #11921, .T. ) ;
#34034=VECTOR ( 'NONE', #31495, 1000.000000000000000 ) ;
#34115=CARTESIAN_POINT ( 'NONE',  ( -11.00000000000000355, 10.00000000000000000, -87.20294101747086302 ) ) ;
#34119=AXIS2_PLACEMENT_3D ( 'NONE', #11338, #31114, #27920 ) ;
#34123=CARTESIAN_POINT ( 'NONE',  ( -45.00000000000002132, 10.00000000000000000, 55.00000000000002132 ) ) ;
#34141=VECTOR ( 'NONE', #19799, 1000.000000000000000 ) ;
#34148=ADVANCED_FACE ( 'NONE', ( #831 ), #31731, .T. ) ;
#34181=LINE ( 'NONE', #24834, #6526 ) ;
#34193=CARTESIAN_POINT ( 'NONE',  ( 40.50000000000000711, 10.00099999999999945, 40.00000000000002842 ) ) ;
#34212=LINE ( 'NONE', #27829, #23070 ) ;
#34218=EDGE_LOOP ( 'NONE', ( #33921, #18429, #24867, #1172, #3365, #23404, #36628, #1318, #28865, #9486, #33432, #14911, #10899, #25062, #24396, #11515 ) ) ;
#34252=( NAMED_UNIT ( * ) PLANE_ANGLE_UNIT ( ) SI_UNIT ( $, .RADIAN. ) );
#34256=DIRECTION ( 'NONE',  ( 0.000000000000000000, 0.000000000000000000, -1.000000000000000000 ) ) ;
#34268=ORIENTED_EDGE ( 'NONE', *, *, #20902, .T. ) ;
#34277=DIRECTION ( 'NONE',  ( -0.000000000000000000, -1.000000000000000000, 0.000000000000000000 ) ) ;
#34286=CARTESIAN_POINT ( 'NONE',  ( -44.99999999999998579, 2.499999999999999556, -60.00000000000000000 ) ) ;
#34309=AXIS2_PLACEMENT_3D ( 'NONE', #34193, #3741, #6097 ) ;
#34332=ORIENTED_EDGE ( 'NONE', *, *, #27177, .T. ) ;
#34361=CYLINDRICAL_SURFACE ( 'NONE', #21219, 10.00000000000000178 ) ;
#34411=EDGE_CURVE ( 'NONE', #38216, #13199, #37399, .T. ) ;
#34428=ORIENTED_EDGE ( 'NONE', *, *, #26578, .T. ) ;
#34433=ORIENTED_EDGE ( 'NONE', *, *, #14771, .T. ) ;
#34457=( NAMED_UNIT ( * ) SI_UNIT ( $, .STERADIAN. ) SOLID_ANGLE_UNIT ( ) );
#34471=CARTESIAN_POINT ( 'NONE',  ( -62.00000000000001421, -2.499999999999999556, -49.99999999999998579 ) ) ;
#34486=EDGE_CURVE ( 'NONE', #19396, #18848, #13975, .T. ) ;
#34493=DIRECTION ( 'NONE',  ( 0.000000000000000000, 0.000000000000000000, -1.000000000000000000 ) ) ;
#34511=CARTESIAN_POINT ( 'NONE',  ( -45.00000000000002132, 2.499999999999999556, -55.00000000000000000 ) ) ;
#34518=CARTESIAN_POINT ( 'NONE',  ( 52.00000000000002842, 2.499999999999999556, 50.00000000000001421 ) ) ;
#34546=DIRECTION ( 'NONE',  ( 0.000000000000000000, -1.734723475976806108E-16, 1.000000000000000000 ) ) ;
#34548=AXIS2_PLACEMENT_3D ( 'NONE', #10938, #1366, #23922 ) ;
#34563=CARTESIAN_POINT ( 'NONE',  ( -45.00000000000002132, 10.00000000000000000, 55.00000000000002132 ) ) ;
#34578=LINE ( 'NONE', #12028, #9655 ) ;
#34586=ADVANCED_FACE ( 'NONE', ( #38018 ), #12279, .F. ) ;
#34595=ORIENTED_EDGE ( 'NONE', *, *, #11268, .T. ) ;
#34604=EDGE_LOOP ( 'NONE', ( #16950, #23919, #29762, #15553, #33715, #30828, #36138, #34595 ) ) ;
#34630=DIRECTION ( 'NONE',  ( 0.000000000000000000, 1.000000000000000000, -0.000000000000000000 ) ) ;
#34639=ORIENTED_EDGE ( 'NONE', *, *, #28765, .T. ) ;
#34644=AXIS2_PLACEMENT_3D ( 'NONE', #1442, #21001, #17812 ) ;
#34667=CARTESIAN_POINT ( 'NONE',  ( -50.00000000000001421, -4.500000000000000000, 36.00000000000002842 ) ) ;
#34671=DIRECTION ( 'NONE',  ( 0.000000000000000000, 0.000000000000000000, 1.000000000000000000 ) ) ;
#34700=CARTESIAN_POINT ( 'NONE',  ( 33.00000000000001421, 8.000000000000000000, 50.00000000000002842 ) ) ;
#34772=DIRECTION ( 'NONE',  ( -0.000000000000000000, -0.000000000000000000, 1.000000000000000000 ) ) ;
#34789=AXIS2_PLACEMENT_3D ( 'NONE', #4626, #33560, #30360 ) ;
#34805=DIRECTION ( 'NONE',  ( 0.000000000000000000, 0.000000000000000000, -1.000000000000000000 ) ) ;
#34806=ORIENTED_EDGE ( 'NONE', *, *, #33398, .T. ) ;
#34807=CARTESIAN_POINT ( 'NONE',  ( -50.00000000000001421, 10.00000000000000000, -59.99999999999999289 ) ) ;
#34816=ORIENTED_EDGE ( 'NONE', *, *, #17092, .T. ) ;
#34830=ORIENTED_EDGE ( 'NONE', *, *, #11873, .T. ) ;
#34833=DIRECTION ( 'NONE',  ( -1.000000000000000000, 0.000000000000000000, 0.000000000000000000 ) ) ;
#34844=EDGE_LOOP ( 'NONE', ( #25024, #41702, #18331, #12985 ) ) ;
#34845=DIRECTION ( 'NONE',  ( 0.000000000000000000, -1.000000000000000000, 0.000000000000000000 ) ) ;
#34849=CIRCLE ( 'NONE', #19908, 4.999999999999997335 ) ;
#34867=ADVANCED_FACE ( 'NONE', ( #29270 ), #32889, .T. ) ;
#34887=ORIENTED_EDGE ( 'NONE', *, *, #14472, .T. ) ;
#34897=VERTEX_POINT ( 'NONE', #564 ) ;
#34900=DIRECTION ( 'NONE',  ( 0.000000000000000000, 0.000000000000000000, 1.000000000000000000 ) ) ;
#34906=CARTESIAN_POINT ( 'NONE',  ( 11.00000000000000355, 26.00000000000000355, -59.99999999999999289 ) ) ;
#34955=ORIENTED_EDGE ( 'NONE', *, *, #9381, .F. ) ;
#34968=AXIS2_PLACEMENT_3D ( 'NONE', #22302, #35276, #19119 ) ;
#34972=CARTESIAN_POINT ( 'NONE',  ( 44.99999999999998579, 10.00000000000000000, -54.99999999999999289 ) ) ;
#35005=ORIENTED_EDGE ( 'NONE', *, *, #15812, .T. ) ;
#35039=LINE ( 'NONE', #41857, #31900 ) ;
#35143=DIRECTION ( 'NONE',  ( -1.000000000000000000, -0.000000000000000000, -0.000000000000000000 ) ) ;
#35176=DIRECTION ( 'NONE',  ( 0.000000000000000000, 1.000000000000000000, 0.000000000000000000 ) ) ;
#35219=LINE ( 'NONE', #18222, #39572 ) ;
#35220=DIRECTION ( 'NONE',  ( -0.000000000000000000, 1.000000000000000000, -0.000000000000000000 ) ) ;
#35276=DIRECTION ( 'NONE',  ( 1.000000000000000000, -0.000000000000000000, -1.067522139062650178E-16 ) ) ;
#35281=AXIS2_PLACEMENT_3D ( 'NONE', #12364, #25348, #38307 ) ;
#35393=CARTESIAN_POINT ( 'NONE',  ( -33.00000000000001421, -4.500000000000000000, 30.00000000000002842 ) ) ;
#35408=DIRECTION ( 'NONE',  ( -0.000000000000000000, -1.000000000000000000, 0.000000000000000000 ) ) ;
#35412=EDGE_LOOP ( 'NONE', ( #9592, #25116, #11706, #29720, #19672, #26129, #32703, #19574 ) ) ;
#35423=EDGE_LOOP ( 'NONE', ( #24781, #40035, #9706, #21218 ) ) ;
#35426=ORIENTED_EDGE ( 'NONE', *, *, #10009, .F. ) ;
#35430=VERTEX_POINT ( 'NONE', #37889 ) ;
#35447=EDGE_CURVE ( 'NONE', #16482, #20097, #27896, .T. ) ;
#35458=DIRECTION ( 'NONE',  ( -1.000000000000000000, -0.000000000000000000, -0.000000000000000000 ) ) ;
#35489=EDGE_LOOP ( 'NONE', ( #2246, #27990, #20201, #34433, #25712, #33493, #28933, #17081 ) ) ;
#35522=VECTOR ( 'NONE', #7023, 1000.000000000000000 ) ;
#35537=DIRECTION ( 'NONE',  ( 0.000000000000000000, 0.000000000000000000, -1.000000000000000000 ) ) ;
#35556=LINE ( 'NONE', #19183, #40945 ) ;
#35572=ORIENTED_EDGE ( 'NONE', *, *, #35447, .F. ) ;
#35582=AXIS2_PLACEMENT_3D ( 'NONE', #30728, #7131, #39877 ) ;
#35634=DIRECTION ( 'NONE',  ( 1.000000000000000000, -0.000000000000000000, 0.000000000000000000 ) ) ;
#35704=AXIS2_PLACEMENT_3D ( 'NONE', #20824, #20397, #4651 ) ;
#35715=DIRECTION ( 'NONE',  ( 0.000000000000000000, 0.000000000000000000, -1.000000000000000000 ) ) ;
#35740=ORIENTED_EDGE ( 'NONE', *, *, #25714, .T. ) ;
#35746=CYLINDRICAL_SURFACE ( 'NONE', #14483, 10.00000000000000178 ) ;
#35749=EDGE_LOOP ( 'NONE', ( #25452, #17856, #22539, #39874, #19943, #36738 ) ) ;
#35750=ORIENTED_EDGE ( 'NONE', *, *, #28362, .T. ) ;
#35753=ORIENTED_EDGE ( 'NONE', *, *, #16861, .F. ) ;
#35797=LINE ( 'NONE', #25402, #32246 ) ;
#35821=LINE ( 'NONE', #9895, #22432 ) ;
#35836=PRODUCT_CONTEXT ( 'NONE', #5173, 'mechanical' ) ;
#35847=VERTEX_POINT ( 'NONE', #9600 ) ;
#35853=CARTESIAN_POINT ( 'NONE',  ( -52.00000000000001421, 2.499999999999999556, -49.99999999999998579 ) ) ;
#35890=AXIS2_PLACEMENT_3D ( 'NONE', #1578, #14127, #20727 ) ;
#35896=EDGE_LOOP ( 'NONE', ( #34955, #23616, #37582, #3820 ) ) ;
#35906=VECTOR ( 'NONE', #14216, 1000.000000000000000 ) ;
#35925=EDGE_CURVE ( 'NONE', #5870, #11057, #25558, .T. ) ;
#35936=DIRECTION ( 'NONE',  ( -1.000000000000000000, -0.000000000000000000, -0.000000000000000000 ) ) ;
#35943=CARTESIAN_POINT ( 'NONE',  ( -52.00000000000001421, 2.499999999999999556, -49.99999999999998579 ) ) ;
#35948=ORIENTED_EDGE ( 'NONE', *, *, #11786, .F. ) ;
#36002=CARTESIAN_POINT ( 'NONE',  ( -33.00000000000001421, 7.999999999999996447, 50.00000000000002842 ) ) ;
#36003=VECTOR ( 'NONE', #40983, 1000.000000000000000 ) ;
#36011=CYLINDRICAL_SURFACE ( 'NONE', #36755, 4.999999999999997335 ) ;
#36046=CARTESIAN_POINT ( 'NONE',  ( -50.00000000000001421, -2.499999999999999556, 36.53589838486226427 ) ) ;
#36076=DIRECTION ( 'NONE',  ( -1.000000000000000000, -0.000000000000000000, -0.000000000000000000 ) ) ;
#36077=CARTESIAN_POINT ( 'NONE',  ( 49.99999999999998579, -10.00000000000000000, 60.00000000000002132 ) ) ;
#36083=DIRECTION ( 'NONE',  ( -0.000000000000000000, 0.000000000000000000, -1.000000000000000000 ) ) ;
#36091=LINE ( 'NONE', #23764, #1495 ) ;
#36095=CARTESIAN_POINT ( 'NONE',  ( -50.00000000000001421, 10.00000000000000000, 55.00000000000002132 ) ) ;
#36134=CARTESIAN_POINT ( 'NONE',  ( 44.99999999999999289, -10.00000000000000000, 55.00000000000002132 ) ) ;
#36138=ORIENTED_EDGE ( 'NONE', *, *, #20902, .F. ) ;
#36151=CARTESIAN_POINT ( 'NONE',  ( -10.00000000000000178, 10.00000000000000000, -87.20294101747086302 ) ) ;
#36160=AXIS2_PLACEMENT_3D ( 'NONE', #11176, #33924, #37129 ) ;
#36192=EDGE_CURVE ( 'NONE', #32443, #4822, #34181, .T. ) ;
#36199=CIRCLE ( 'NONE', #9718, 4.000000000000003553 ) ;
#36211=LINE ( 'NONE', #36002, #14920 ) ;
#36242=CARTESIAN_POINT ( 'NONE',  ( -48.00000000000001421, -4.500000000000000000, 40.00000000000002842 ) ) ;
#36256=ORIENTED_EDGE ( 'NONE', *, *, #5879, .T. ) ;
#36284=CARTESIAN_POINT ( 'NONE',  ( -50.00000000000001421, -10.00000000000000000, 60.00000000000002132 ) ) ;
#36302=CARTESIAN_POINT ( 'NONE',  ( 44.99999999999998579, -10.00000000000000000, -54.99999999999999289 ) ) ;
#36353=CARTESIAN_POINT ( 'NONE',  ( 44.99999999999998579, 10.00000000000000000, 60.00000000000002132 ) ) ;
#36363=AXIS2_PLACEMENT_3D ( 'NONE', #38903, #9781, #35715 ) ;
#36365=EDGE_CURVE ( 'NONE', #12609, #14520, #38206, .T. ) ;
#36369=EDGE_LOOP ( 'NONE', ( #6654, #38041, #40763, #23415 ) ) ;
#36371=AXIS2_PLACEMENT_3D ( 'NONE', #28441, #12064, #6108 ) ;
#36388=CARTESIAN_POINT ( 'NONE',  ( 43.49958017181736381, -8.499685129138665474, 40.21211302601980009 ) ) ;
#36416=EDGE_CURVE ( 'NONE', #26597, #40855, #21485, .T. ) ;
#36460=CARTESIAN_POINT ( 'NONE',  ( 38.52390716863592957, -7.800592889815003872, 42.26512378391644376 ) ) ;
#36476=CYLINDRICAL_SURFACE ( 'NONE', #17854, 3.000000000000002665 ) ;
#36485=DIRECTION ( 'NONE',  ( 1.000000000000000000, -0.000000000000000000, -0.000000000000000000 ) ) ;
#36525=ORIENTED_EDGE ( 'NONE', *, *, #24140, .F. ) ;
#36574=LINE ( 'NONE', #11054, #28156 ) ;
#36628=ORIENTED_EDGE ( 'NONE', *, *, #20185, .F. ) ;
#36633=EDGE_LOOP ( 'NONE', ( #9849, #27014, #3502, #11673 ) ) ;
#36639=CARTESIAN_POINT ( 'NONE',  ( 11.00000000000000355, 26.00000000000000355, 60.00000000000002132 ) ) ;
#36650=DIRECTION ( 'NONE',  ( 1.000000000000000000, 0.000000000000000000, 0.000000000000000000 ) ) ;
#36654=ADVANCED_FACE ( 'NONE', ( #9115 ), #15719, .T. ) ;
#36692=VERTEX_POINT ( 'NONE', #5295 ) ;
#36708=LINE ( 'NONE', #33737, #8487 ) ;
#36738=ORIENTED_EDGE ( 'NONE', *, *, #20167, .T. ) ;
#36754=LINE ( 'NONE', #14004, #12181 ) ;
#36755=AXIS2_PLACEMENT_3D ( 'NONE', #29415, #13465, #19639 ) ;
#36757=CYLINDRICAL_SURFACE ( 'NONE', #17309, 3.000000000000002665 ) ;
#36810=VERTEX_POINT ( 'NONE', #39507 ) ;
#36813=VECTOR ( 'NONE', #5895, 1000.000000000000000 ) ;
#36819=CARTESIAN_POINT ( 'NONE',  ( 43.08447751878441068, -8.197737767270092846, 38.46464586805510777 ) ) ;
#36843=ORIENTED_EDGE ( 'NONE', *, *, #3799, .F. ) ;
#36891=CARTESIAN_POINT ( 'NONE',  ( 37.66885629351435227, -8.374584989461757445, 38.98823203435226503 ) ) ;
#36908=CARTESIAN_POINT ( 'NONE',  ( -45.00000000000002132, 2.499999999999999556, 60.00000000000002132 ) ) ;
#36971=DIRECTION ( 'NONE',  ( -1.000000000000000000, -0.000000000000000000, -0.000000000000000000 ) ) ;
#37044=CARTESIAN_POINT ( 'NONE',  ( -45.00000000000002132, 2.499999999999999556, 55.00000000000002132 ) ) ;
#37070=ORIENTED_EDGE ( 'NONE', *, *, #14749, .F. ) ;
#37109=CARTESIAN_POINT ( 'NONE',  ( 40.08990668953756398, -7.170509413432503365, 37.02142031418924262 ) ) ;
#37122=DIRECTION ( 'NONE',  ( 0.000000000000000000, -1.000000000000000000, 0.000000000000000000 ) ) ;
#37129=DIRECTION ( 'NONE',  ( 0.000000000000000000, 0.000000000000000000, -1.000000000000000000 ) ) ;
#37134=CARTESIAN_POINT ( 'NONE',  ( -33.00000000000001421, 8.000000000000000000, 30.00000000000002132 ) ) ;
#37140=LINE ( 'NONE', #30532, #30914 ) ;
#37253=EDGE_CURVE ( 'NONE', #29490, #3926, #2895, .T. ) ;
#37280=EDGE_CURVE ( 'NONE', #40859, #11983, #32835, .T. ) ;
#37304=VERTEX_POINT ( 'NONE', #36046 ) ;
#37309=CARTESIAN_POINT ( 'NONE',  ( 39.15228859180873400, -7.464796833660714448, 37.31285029933195574 ) ) ;
#37343=CARTESIAN_POINT ( 'NONE',  ( -11.00000000000000355, 10.00000000000000000, 60.00000000000002132 ) ) ;
#37353=ORIENTED_EDGE ( 'NONE', *, *, #20234, .F. ) ;
#37360=CARTESIAN_POINT ( 'NONE',  ( 49.99999999999998579, -2.499999999999999556, 55.00000000000002132 ) ) ;
#37367=ORIENTED_EDGE ( 'NONE', *, *, #1262, .F. ) ;
#37389=FACE_OUTER_BOUND ( 'NONE', #30731, .T. ) ;
#37399=LINE ( 'NONE', #4854, #12599 ) ;
#37424=EDGE_CURVE ( 'NONE', #11057, #41722, #13840, .T. ) ;
#37441=CARTESIAN_POINT ( 'NONE',  ( 49.99999999999998579, 10.00000000000000000, 55.00000000000002132 ) ) ;
#37461=VERTEX_POINT ( 'NONE', #36908 ) ;
#37469=VERTEX_POINT ( 'NONE', #23515 ) ;
#37476=VERTEX_POINT ( 'NONE', #11170 ) ;
#37482=LINE ( 'NONE', #2378, #41079 ) ;
#37495=CARTESIAN_POINT ( 'NONE',  ( -10.00000000000000178, 10.00000000000000000, 60.00000000000002132 ) ) ;
#37536=FACE_OUTER_BOUND ( 'NONE', #29341, .T. ) ;
#37550=LINE ( 'NONE', #14800, #17821 ) ;
#37581=VECTOR ( 'NONE', #5421, 1000.000000000000000 ) ;
#37582=ORIENTED_EDGE ( 'NONE', *, *, #25665, .T. ) ;
#37584=VECTOR ( 'NONE', #10430, 1000.000000000000000 ) ;
#37612=CARTESIAN_POINT ( 'NONE',  ( -45.00000000000002132, -2.500000000000000444, 60.00000000000002132 ) ) ;
#37619=EDGE_CURVE ( 'NONE', #39773, #27620, #30229, .T. ) ;
#37622=CIRCLE ( 'NONE', #30152, 4.999999999999997335 ) ;
#37626=EDGE_LOOP ( 'NONE', ( #21354, #25809, #16764, #5028, #29349 ) ) ;
#37631=VECTOR ( 'NONE', #22332, 1000.000000000000000 ) ;
#37641=ADVANCED_FACE ( 'NONE', ( #1104 ), #6834, .F. ) ;
#37644=DIRECTION ( 'NONE',  ( 0.000000000000000000, 0.000000000000000000, -1.000000000000000000 ) ) ;
#37648=DIRECTION ( 'NONE',  ( -1.000000000000000000, 0.000000000000000000, 0.000000000000000000 ) ) ;
#37712=LINE ( 'NONE', #33297, #17538 ) ;
#37745=FACE_OUTER_BOUND ( 'NONE', #2681, .T. ) ;
#37756=CARTESIAN_POINT ( 'NONE',  ( 44.99999999999998579, 10.00000000000000000, -54.99999999999999289 ) ) ;
#37758=DIRECTION ( 'NONE',  ( -1.000000000000000000, -0.000000000000000000, -0.000000000000000000 ) ) ;
#37769=VERTEX_POINT ( 'NONE', #34667 ) ;
#37799=ORIENTED_EDGE ( 'NONE', *, *, #27440, .T. ) ;
#37810=FACE_OUTER_BOUND ( 'NONE', #33491, .T. ) ;
#37843=EDGE_CURVE ( 'NONE', #37461, #27592, #19955, .T. ) ;
#37845=EDGE_CURVE ( 'NONE', #6074, #38231, #37622, .T. ) ;
#37879=CARTESIAN_POINT ( 'NONE',  ( 62.00000000000001421, -2.499999999999999556, -60.00000000000000000 ) ) ;
#37880=ORIENTED_EDGE ( 'NONE', *, *, #25463, .T. ) ;
#37889=CARTESIAN_POINT ( 'NONE',  ( -48.00000000000001421, -10.00000000000000000, 55.00000000000002132 ) ) ;
#37925=ORIENTED_EDGE ( 'NONE', *, *, #34486, .F. ) ;
#37929=CARTESIAN_POINT ( 'NONE',  ( 49.99999999999998579, 10.00000000000000000, 60.00000000000002132 ) ) ;
#37931=DIRECTION ( 'NONE',  ( 0.000000000000000000, 0.000000000000000000, 1.000000000000000000 ) ) ;
#37934=FACE_OUTER_BOUND ( 'NONE', #41765, .T. ) ;
#37937=EDGE_CURVE ( 'NONE', #27676, #4135, #21901, .T. ) ;
#37945=LINE ( 'NONE', #28576, #23143 ) ;
#37950=VECTOR ( 'NONE', #10160, 1000.000000000000000 ) ;
#37990=ORIENTED_EDGE ( 'NONE', *, *, #40187, .F. ) ;
#38018=FACE_OUTER_BOUND ( 'NONE', #18105, .T. ) ;
#38036=EDGE_LOOP ( 'NONE', ( #18962, #2479 ) ) ;
#38041=ORIENTED_EDGE ( 'NONE', *, *, #2725, .T. ) ;
#38046=VECTOR ( 'NONE', #21617, 1000.000000000000000 ) ;
#38081=VECTOR ( 'NONE', #40303, 1000.000000000000000 ) ;
#38083=VERTEX_POINT ( 'NONE', #36353 ) ;
#38093=ADVANCED_FACE ( 'NONE', ( #29325 ), #7003, .T. ) ;
#38095=CARTESIAN_POINT ( 'NONE',  ( -45.00000000000002132, -10.00000000000000000, 55.00000000000002132 ) ) ;
#38183=FACE_OUTER_BOUND ( 'NONE', #25976, .T. ) ;
#38192=EDGE_LOOP ( 'NONE', ( #18796, #15880 ) ) ;
#38198=ORIENTED_EDGE ( 'NONE', *, *, #5913, .T. ) ;
#38206=LINE ( 'NONE', #34807, #38471 ) ;
#38216=VERTEX_POINT ( 'NONE', #37612 ) ;
#38231=VERTEX_POINT ( 'NONE', #20832 ) ;
#38283=EDGE_LOOP ( 'NONE', ( #32170, #7344, #14880, #13449 ) ) ;
#38297=AXIS2_PLACEMENT_3D ( 'NONE', #16132, #3142, #36083 ) ;
#38304=DIRECTION ( 'NONE',  ( -0.000000000000000000, -0.000000000000000000, 1.000000000000000000 ) ) ;
#38307=DIRECTION ( 'NONE',  ( 0.000000000000000000, 0.000000000000000000, -1.000000000000000000 ) ) ;
#38333=ORIENTED_EDGE ( 'NONE', *, *, #25177, .F. ) ;
#38355=ORIENTED_EDGE ( 'NONE', *, *, #38952, .T. ) ;
#38412=ORIENTED_EDGE ( 'NONE', *, *, #25714, .F. ) ;
#38415=ADVANCED_FACE ( 'NONE', ( #15288 ), #28870, .T. ) ;
#38470=CARTESIAN_POINT ( 'NONE',  ( 44.99999999999999289, 2.499999999999999556, 55.00000000000002132 ) ) ;
#38471=VECTOR ( 'NONE', #5675, 1000.000000000000000 ) ;
#38473=CARTESIAN_POINT ( 'NONE',  ( 49.99999999999998579, 10.00000000000000000, -55.00000000000000000 ) ) ;
#38541=DIRECTION ( 'NONE',  ( -1.000000000000000000, 0.000000000000000000, -0.000000000000000000 ) ) ;
#38551=ORIENTED_EDGE ( 'NONE', *, *, #22155, .F. ) ;
#38586=DIRECTION ( 'NONE',  ( 0.000000000000000000, 0.000000000000000000, -1.000000000000000000 ) ) ;
#38589=EDGE_CURVE ( 'NONE', #41543, #14520, #25904, .T. ) ;
#38610=EDGE_CURVE ( 'NONE', #31393, #1025, #16545, .T. ) ;
#38619=VERTEX_POINT ( 'NONE', #20354 ) ;
#38622=CARTESIAN_POINT ( 'NONE',  ( -45.00000000000002132, 10.00000000000000000, -55.00000000000000000 ) ) ;
#38623=CARTESIAN_POINT ( 'NONE',  ( -52.00000000000001421, 10.00000000000000000, -59.99999999999999289 ) ) ;
#38649=DIRECTION ( 'NONE',  ( -1.000000000000000000, 0.000000000000000000, 0.000000000000000000 ) ) ;
#38674=ORIENTED_EDGE ( 'NONE', *, *, #38589, .T. ) ;
#38684=AXIS2_PLACEMENT_3D ( 'NONE', #26443, #16458, #29408 ) ;
#38711=CIRCLE ( 'NONE', #6767, 3.000000000000002665 ) ;
#38735=ORIENTED_EDGE ( 'NONE', *, *, #24140, .T. ) ;
#38759=LINE ( 'NONE', #29377, #19757 ) ;
#38786=DIRECTION ( 'NONE',  ( 0.000000000000000000, 0.000000000000000000, -1.000000000000000000 ) ) ;
#38860=AXIS2_PLACEMENT_3D ( 'NONE', #34563, #17987, #40735 ) ;
#38865=PLANE ( 'NONE',  #38297 ) ;
#38903=CARTESIAN_POINT ( 'NONE',  ( -50.00000000000001421, -4.500000000000000000, 40.00000000000002842 ) ) ;
#38921=AXIS2_PLACEMENT_3D ( 'NONE', #912, #17074, #20261 ) ;
#38922=LINE ( 'NONE', #33161, #15181 ) ;
#38931=ORIENTED_EDGE ( 'NONE', *, *, #16859, .F. ) ;
#38952=EDGE_CURVE ( 'NONE', #1211, #21502, #18629, .T. ) ;
#38981=VECTOR ( 'NONE', #23558, 1000.000000000000000 ) ;
#39028=ORIENTED_EDGE ( 'NONE', *, *, #34411, .T. ) ;
#39038=CIRCLE ( 'NONE', #7779, 4.000000000000003553 ) ;
#39054=CARTESIAN_POINT ( 'NONE',  ( -11.00000000000000355, 10.00000000000000000, 60.00000000000002132 ) ) ;
#39062=DIRECTION ( 'NONE',  ( 0.000000000000000000, -5.551115123125782702E-16, -1.000000000000000000 ) ) ;
#39075=LINE ( 'NONE', #26745, #27241 ) ;
#39076=DIRECTION ( 'NONE',  ( -0.000000000000000000, 1.000000000000000000, -0.000000000000000000 ) ) ;
#39080=DIRECTION ( 'NONE',  ( 0.000000000000000000, 0.000000000000000000, -1.000000000000000000 ) ) ;
#39093=CARTESIAN_POINT ( 'NONE',  ( -62.00000000000002842, -2.499999999999999556, 50.00000000000001421 ) ) ;
#39097=CARTESIAN_POINT ( 'NONE',  ( 44.99999999999998579, 8.000000000000000000, -57.99999999999998579 ) ) ;
#39124=ORIENTED_EDGE ( 'NONE', *, *, #26578, .F. ) ;
#39130=LINE ( 'NONE', #9594, #1380 ) ;
#39229=EDGE_CURVE ( 'NONE', #1429, #38619, #25421, .T. ) ;
#39241=DIRECTION ( 'NONE',  ( 0.000000000000000000, 0.000000000000000000, 1.000000000000000000 ) ) ;
#39267=DIRECTION ( 'NONE',  ( 0.000000000000000000, 0.000000000000000000, -1.000000000000000000 ) ) ;
#39274=DIRECTION ( 'NONE',  ( 1.000000000000000000, 0.000000000000000000, 0.000000000000000000 ) ) ;
#39306=DIRECTION ( 'NONE',  ( 0.000000000000000000, 0.000000000000000000, -1.000000000000000000 ) ) ;
#39310=CARTESIAN_POINT ( 'NONE',  ( -45.00000000000002132, -2.499999999999999556, -55.00000000000000000 ) ) ;
#39331=VERTEX_POINT ( 'NONE', #29865 ) ;
#39337=ADVANCED_FACE ( 'NONE', ( #23499 ), #32430, .F. ) ;
#39349=CARTESIAN_POINT ( 'NONE',  ( 43.39717995588247845, -8.423377063002785547, 39.19476686319822534 ) ) ;
#39354=CARTESIAN_POINT ( 'NONE',  ( 33.00000000000001421, -10.00000000000000000, 40.00000000000002842 ) ) ;
#39379=ORIENTED_EDGE ( 'NONE', *, *, #29406, .T. ) ;
#39389=ORIENTED_EDGE ( 'NONE', *, *, #26291, .T. ) ;
#39460=EDGE_CURVE ( 'NONE', #40855, #9283, #39038, .T. ) ;
#39467=AXIS2_PLACEMENT_3D ( 'NONE', #6046, #2857, #19024 ) ;
#39471=CARTESIAN_POINT ( 'NONE',  ( -45.00000000000002132, 10.00000000000000000, 60.00000000000002132 ) ) ;
#39473=CARTESIAN_POINT ( 'NONE',  ( -9.999999999999998224, 25.00000000000000000, 60.00000000000002132 ) ) ;
#39490=DIRECTION ( 'NONE',  ( 0.000000000000000000, -1.000000000000000000, 0.000000000000000000 ) ) ;
#39497=LINE ( 'NONE', #36095, #37950 ) ;
#39507=CARTESIAN_POINT ( 'NONE',  ( -50.00000000000001421, -2.500000000000000444, 55.00000000000002132 ) ) ;
#39560=ORIENTED_EDGE ( 'NONE', *, *, #17065, .T. ) ;
#39572=VECTOR ( 'NONE', #12681, 1000.000000000000000 ) ;
#39595=CARTESIAN_POINT ( 'NONE',  ( 33.00000000000001421, -4.500000000000000000, 40.00000000000002842 ) ) ;
#39606=ORIENTED_EDGE ( 'NONE', *, *, #3807, .F. ) ;
#39643=EDGE_CURVE ( 'NONE', #35847, #40514, #20685, .T. ) ;
#39645=CARTESIAN_POINT ( 'NONE',  ( 38.52672849965874491, -7.798910822842188395, 37.73247971346996366 ) ) ;
#39655=ORIENTED_EDGE ( 'NONE', *, *, #12235, .T. ) ;
#39660=FACE_OUTER_BOUND ( 'NONE', #36633, .T. ) ;
#39773=VERTEX_POINT ( 'NONE', #23329 ) ;
#39786=ORIENTED_EDGE ( 'NONE', *, *, #22772, .F. ) ;
#39787=ORIENTED_EDGE ( 'NONE', *, *, #28362, .F. ) ;
#39794=CARTESIAN_POINT ( 'NONE',  ( 41.30658877145464913, -7.259278429453377868, 42.89655275347914198 ) ) ;
#39829=EDGE_CURVE ( 'NONE', #40914, #41076, #20135, .T. ) ;
#39874=ORIENTED_EDGE ( 'NONE', *, *, #30364, .T. ) ;
#39875=ORIENTED_EDGE ( 'NONE', *, *, #8933, .F. ) ;
#39877=DIRECTION ( 'NONE',  ( 0.000000000000000000, 0.000000000000000000, 1.000000000000000000 ) ) ;
#39889=DIRECTION ( 'NONE',  ( 0.000000000000000000, 0.000000000000000000, -1.000000000000000000 ) ) ;
#39896=DIRECTION ( 'NONE',  ( 1.000000000000000000, -0.000000000000000000, -0.000000000000000000 ) ) ;
#39913=ORIENTED_EDGE ( 'NONE', *, *, #3807, .T. ) ;
#39961=CARTESIAN_POINT ( 'NONE',  ( -50.00000000000001421, 10.00000000000000000, -59.99999999999999289 ) ) ;
#39981=ORIENTED_EDGE ( 'NONE', *, *, #14944, .T. ) ;
#39985=PLANE ( 'NONE',  #30080 ) ;
#39991=ORIENTED_EDGE ( 'NONE', *, *, #19885, .T. ) ;
#40000=CARTESIAN_POINT ( 'NONE',  ( 42.32990480731965732, -7.714196927292076289, 42.38474217628819218 ) ) ;
#40012=ADVANCED_FACE ( 'NONE', ( #25583 ), #28961, .T. ) ;
#40030=AXIS2_PLACEMENT_3D ( 'NONE', #40625, #37648, #14891 ) ;
#40035=ORIENTED_EDGE ( 'NONE', *, *, #27440, .F. ) ;
#40068=VERTEX_POINT ( 'NONE', #6427 ) ;
#40072=CARTESIAN_POINT ( 'NONE',  ( 37.52264654860105253, -8.482944780242485550, 39.57985533149818025 ) ) ;
#40078=AXIS2_PLACEMENT_3D ( 'NONE', #15910, #15060, #12276 ) ;
#40081=ORIENTED_EDGE ( 'NONE', *, *, #28713, .T. ) ;
#40087=VECTOR ( 'NONE', #34900, 1000.000000000000000 ) ;
#40104=CIRCLE ( 'NONE', #21767, 3.000000000000002665 ) ;
#40154=CARTESIAN_POINT ( 'NONE',  ( 44.99999999999998579, -2.500000000000000444, 60.00000000000002132 ) ) ;
#40187=EDGE_CURVE ( 'NONE', #40353, #24557, #22173, .T. ) ;
#40241=CARTESIAN_POINT ( 'NONE',  ( -11.00000000000000355, 10.00000000000000000, -87.20294101747086302 ) ) ;
#40294=ORIENTED_EDGE ( 'NONE', *, *, #11391, .T. ) ;
#40298=ORIENTED_EDGE ( 'NONE', *, *, #10920, .T. ) ;
#40303=DIRECTION ( 'NONE',  ( 0.000000000000000000, -1.000000000000000000, 0.000000000000000000 ) ) ;
#40305=ORIENTED_EDGE ( 'NONE', *, *, #30067, .F. ) ;
#40319=VECTOR ( 'NONE', #14398, 1000.000000000000000 ) ;
#40353=VERTEX_POINT ( 'NONE', #5201 ) ;
#40357=VERTEX_POINT ( 'NONE', #15414 ) ;
#40363=EDGE_CURVE ( 'NONE', #33660, #25504, #11782, .T. ) ;
#40439=EDGE_CURVE ( 'NONE', #21965, #29446, #35797, .T. ) ;
#40442=AXIS2_PLACEMENT_3D ( 'NONE', #11131, #24112, #36650 ) ;
#40444=PRODUCT ( 'Main Plastic Part', 'Main Plastic Part', '', ( #35836 ) ) ;
#40462=FACE_OUTER_BOUND ( 'NONE', #15082, .T. ) ;
#40508=ORIENTED_EDGE ( 'NONE', *, *, #4634, .F. ) ;
#40510=DIRECTION ( 'NONE',  ( 0.000000000000000000, 0.000000000000000000, -1.000000000000000000 ) ) ;
#40514=VERTEX_POINT ( 'NONE', #17295 ) ;
#40554=ORIENTED_EDGE ( 'NONE', *, *, #10920, .F. ) ;
#40578=DIRECTION ( 'NONE',  ( 0.000000000000000000, 0.000000000000000000, -1.000000000000000000 ) ) ;
#40582=LINE ( 'NONE', #17209, #11583 ) ;
#40604=ORIENTED_EDGE ( 'NONE', *, *, #15812, .F. ) ;
#40605=VERTEX_POINT ( 'NONE', #17505 ) ;
#40625=CARTESIAN_POINT ( 'NONE',  ( 49.99999999999998579, 10.00000000000000000, 60.00000000000002132 ) ) ;
#40658=ORIENTED_EDGE ( 'NONE', *, *, #37843, .F. ) ;
#40659=LINE ( 'NONE', #12359, #13108 ) ;
#40679=CARTESIAN_POINT ( 'NONE',  ( 49.99999999999998579, -2.499999999999999556, 43.46410161513777837 ) ) ;
#40735=DIRECTION ( 'NONE',  ( 0.000000000000000000, 0.000000000000000000, -1.000000000000000000 ) ) ;
#40763=ORIENTED_EDGE ( 'NONE', *, *, #17568, .F. ) ;
#40801=DIRECTION ( 'NONE',  ( 1.000000000000000000, 0.000000000000000000, 0.000000000000000000 ) ) ;
#40805=DIRECTION ( 'NONE',  ( 0.000000000000000000, 0.000000000000000000, -1.000000000000000000 ) ) ;
#40855=VERTEX_POINT ( 'NONE', #14734 ) ;
#40859=VERTEX_POINT ( 'NONE', #11941 ) ;
#40864=CARTESIAN_POINT ( 'NONE',  ( -45.00000000000002132, 10.00000000000000000, -55.00000000000000000 ) ) ;
#40890=EDGE_CURVE ( 'NONE', #41543, #3926, #31509, .T. ) ;
#40905=CARTESIAN_POINT ( 'NONE',  ( 47.99999999999998579, -10.00000000000000000, 31.64835345575499304 ) ) ;
#40914=VERTEX_POINT ( 'NONE', #5151 ) ;
#40928=LINE ( 'NONE', #5622, #7154 ) ;
#40935=CYLINDRICAL_SURFACE ( 'NONE', #23834, 10.00000000000000178 ) ;
#40942=EDGE_CURVE ( 'NONE', #17279, #23938, #41779, .T. ) ;
#40945=VECTOR ( 'NONE', #32561, 1000.000000000000000 ) ;
#40949=VECTOR ( 'NONE', #5744, 1000.000000000000000 ) ;
#40950=DIRECTION ( 'NONE',  ( 0.000000000000000000, 0.000000000000000000, -1.000000000000000000 ) ) ;
#40963=CARTESIAN_POINT ( 'NONE',  ( -11.00000000000000355, 26.00000000000000355, -87.20294101747086302 ) ) ;
#40969=ORIENTED_EDGE ( 'NONE', *, *, #26453, .T. ) ;
#40975=EDGE_CURVE ( 'NONE', #7819, #3291, #37482, .T. ) ;
#40979=LINE ( 'NONE', #13092, #30755 ) ;
#40983=DIRECTION ( 'NONE',  ( 1.000000000000000000, -0.000000000000000000, -1.067522139062650178E-16 ) ) ;
#41023=AXIS2_PLACEMENT_3D ( 'NONE', #4284, #13639, #20665 ) ;
#41025=EDGE_CURVE ( 'NONE', #20613, #37469, #9603, .T. ) ;
#41035=CARTESIAN_POINT ( 'NONE',  ( 33.00000000000001421, -10.00000000000000000, 31.64835345575499304 ) ) ;
#41040=AXIS2_PLACEMENT_3D ( 'NONE', #32281, #8675, #41437 ) ;
#41057=DIRECTION ( 'NONE',  ( -0.000000000000000000, -1.000000000000000000, 0.000000000000000000 ) ) ;
#41076=VERTEX_POINT ( 'NONE', #8963 ) ;
#41079=VECTOR ( 'NONE', #28315, 1000.000000000000000 ) ;
#41114=AXIS2_PLACEMENT_3D ( 'NONE', #37756, #21376, #5635 ) ;
#41127=CARTESIAN_POINT ( 'NONE',  ( 33.00000000000001421, -4.500000000000000000, 40.00000000000002842 ) ) ;
#41128=DIRECTION ( 'NONE',  ( 0.000000000000000000, 0.000000000000000000, 1.000000000000000000 ) ) ;
#41130=CARTESIAN_POINT ( 'NONE',  ( 44.99999999999998579, 2.499999999999999556, -54.99999999999999289 ) ) ;
#41140=ORIENTED_EDGE ( 'NONE', *, *, #8190, .T. ) ;
#41181=DIRECTION ( 'NONE',  ( 0.000000000000000000, 0.000000000000000000, -1.000000000000000000 ) ) ;
#41196=DIRECTION ( 'NONE',  ( -0.000000000000000000, -1.000000000000000000, 0.000000000000000000 ) ) ;
#41290=DIRECTION ( 'NONE',  ( 0.000000000000000000, 0.000000000000000000, -1.000000000000000000 ) ) ;
#41294=LINE ( 'NONE', #8747, #33486 ) ;
#41335=FACE_OUTER_BOUND ( 'NONE', #34844, .T. ) ;
#41347=VERTEX_POINT ( 'NONE', #41035 ) ;
#41404=AXIS2_PLACEMENT_3D ( 'NONE', #26084, #22884, #39241 ) ;
#41418=VECTOR ( 'NONE', #28971, 1000.000000000000000 ) ;
#41420=CARTESIAN_POINT ( 'NONE',  ( -62.00000000000001421, -2.499999999999999556, -60.00000000000000000 ) ) ;
#41437=DIRECTION ( 'NONE',  ( -1.000000000000000000, 0.000000000000000000, -0.000000000000000000 ) ) ;
#41438=CARTESIAN_POINT ( 'NONE',  ( 52.00000000000002132, 2.499999999999999556, -49.99999999999998579 ) ) ;
#41442=CARTESIAN_POINT ( 'NONE',  ( -52.00000000000001421, -2.499999999999999556, -49.99999999999998579 ) ) ;
#41446=ORIENTED_EDGE ( 'NONE', *, *, #22629, .F. ) ;
#41471=ADVANCED_FACE ( 'NONE', ( #9338 ), #31662, .F. ) ;
#41514=CYLINDRICAL_SURFACE ( 'NONE', #35281, 4.000000000000003553 ) ;
#41515=ORIENTED_EDGE ( 'NONE', *, *, #14771, .F. ) ;
#41534=ORIENTED_EDGE ( 'NONE', *, *, #7890, .F. ) ;
#41543=VERTEX_POINT ( 'NONE', #26770 ) ;
#41572=CARTESIAN_POINT ( 'NONE',  ( 44.99999999999998579, 10.00000000000000000, -54.99999999999999289 ) ) ;
#41576=PLANE ( 'NONE',  #24551 ) ;
#41578=VECTOR ( 'NONE', #23744, 1000.000000000000000 ) ;
#41624=VECTOR ( 'NONE', #16424, 1000.000000000000000 ) ;
#41660=STYLED_ITEM('',(#42166),#10332);
#41702=ORIENTED_EDGE ( 'NONE', *, *, #29277, .F. ) ;
#41722=VERTEX_POINT ( 'NONE', #40154 ) ;
#41733=ADVANCED_FACE ( 'NONE', ( #37745 ), #36757, .F. ) ;
#41740=CARTESIAN_POINT ( 'NONE',  ( 10.00000000000000178, 25.00000000000000000, -87.20294101747086302 ) ) ;
#41741=VECTOR ( 'NONE', #24220, 1000.000000000000000 ) ;
#41743=PLANE ( 'NONE',  #12375 ) ;
#41744=ORIENTED_EDGE ( 'NONE', *, *, #27177, .F. ) ;
#41751=DIRECTION ( 'NONE',  ( 0.000000000000000000, -1.000000000000000000, 0.000000000000000000 ) ) ;
#41765=EDGE_LOOP ( 'NONE', ( #40554, #6408, #16612, #17274 ) ) ;
#41768=EDGE_LOOP ( 'NONE', ( #33477, #1024, #11523, #9272, #29729, #38735, #16295, #40298, #37925, #16743, #31195, #39655, #24914, #9274, #9062, #23977 ) ) ;
#41779=CIRCLE ( 'NONE', #32275, 10.00000000000000178 ) ;
#41830=DIRECTION ( 'NONE',  ( 0.000000000000000000, 0.000000000000000000, -1.000000000000000000 ) ) ;
#41857=CARTESIAN_POINT ( 'NONE',  ( -50.00000000000001421, 10.00000000000000000, 60.00000000000002132 ) ) ;
#41873=FACE_OUTER_BOUND ( 'NONE', #37626, .T. ) ;
#41891=ORIENTED_EDGE ( 'NONE', *, *, #15093, .F. ) ;
#42028=CARTESIAN_POINT ( 'NONE',  ( -50.00000000000001421, 10.00000000000000000, 60.00000000000002132 ) ) ;
#42036=CIRCLE ( 'NONE', #23693, 4.999999999999997335 ) ;
#42037=DIRECTION ( 'NONE',  ( -0.000000000000000000, 1.000000000000000000, -0.000000000000000000 ) ) ;
#42055=CARTESIAN_POINT ( 'NONE',  ( -73.31370849898480913, -4.500000000000000000, 36.00000000000002842 ) ) ;
#42060=DIRECTION ( 'NONE',  ( 0.000000000000000000, 0.000000000000000000, 1.000000000000000000 ) ) ;
#42088=EDGE_LOOP ( 'NONE', ( #30359, #38355, #20260, #16042 ) ) ;
#42160=COLOUR_RGB('Off White',0.89,0.88,0.83);
#42161=FILL_AREA_STYLE_COLOUR('',#42160);
#42162=FILL_AREA_STYLE('',(#42161));
#42163=SURFACE_STYLE_FILL_AREA(#42162);
#42164=SURFACE_SIDE_STYLE('',(#42163));
#42165=SURFACE_STYLE_USAGE(.BOTH.,#42164);
#42166=PRESENTATION_STYLE_ASSIGNMENT((#42165));
ENDSEC;
END-ISO-10303-21;
